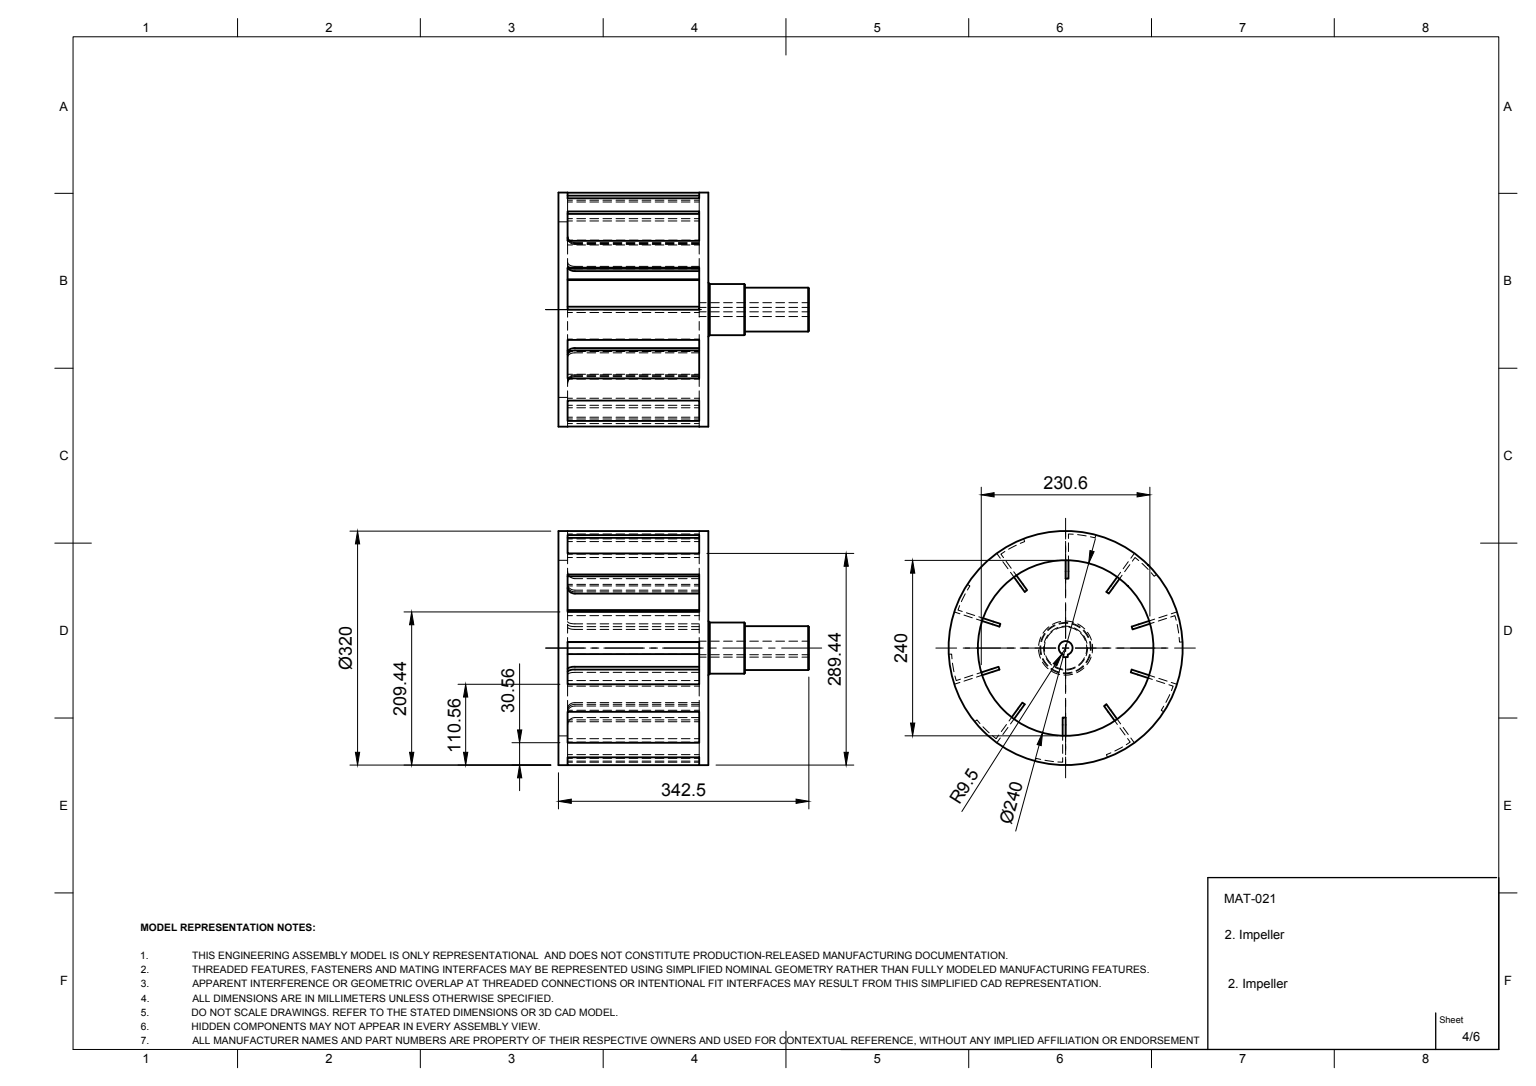
ISO-10303-21;
HEADER;
/* Generated by software containing ST-Developer
 * from STEP Tools, Inc. (www.steptools.com) 
 */

FILE_DESCRIPTION(
/* description */ ('STEP AP214'),
/* implementation_level */ '2;1');

FILE_NAME(
/* name */ '2. Impeller.step',
/* time_stamp */ '2026-11-14T06:27:21-08:00',
/* author */ (''),
/* organization */ (''),
/* preprocessor_version */ 'ST-DEVELOPER v20.2',
/* originating_system */ 'Autodesk Translation Framework v15.17.0.0',
/* authorisation */ '');

FILE_SCHEMA (('AUTOMOTIVE_DESIGN { 1 0 10303 214 3 1 1 }'));
ENDSEC;

DATA;
#10=MECHANICAL_DESIGN_GEOMETRIC_PRESENTATION_REPRESENTATION('',(#36),#27541);
#28=SHAPE_REPRESENTATION_RELATIONSHIP('SRR','None',#27562,#32);
#32=ADVANCED_BREP_SHAPE_REPRESENTATION('',(#63),#27538);
#36=STYLED_ITEM('',(#27591),#63);
#63=MANIFOLD_SOLID_BREP('Body1',#11824);
#248=PLANE('',#12491);
#249=PLANE('',#12492);
#250=PLANE('',#12493);
#251=PLANE('',#12494);
#252=PLANE('',#12495);
#253=PLANE('',#12496);
#254=PLANE('',#12497);
#255=PLANE('',#12498);
#256=PLANE('',#12499);
#257=PLANE('',#12500);
#258=PLANE('',#12501);
#259=PLANE('',#12512);
#260=PLANE('',#12513);
#261=PLANE('',#12514);
#262=PLANE('',#12515);
#263=PLANE('',#12516);
#264=PLANE('',#12520);
#265=PLANE('',#12521);
#266=PLANE('',#12524);
#267=PLANE('',#12525);
#268=PLANE('',#12529);
#269=PLANE('',#12530);
#270=PLANE('',#12532);
#271=PLANE('',#12533);
#272=PLANE('',#12537);
#273=PLANE('',#12538);
#274=PLANE('',#12540);
#275=PLANE('',#12541);
#276=PLANE('',#12545);
#277=PLANE('',#12546);
#278=PLANE('',#12548);
#279=PLANE('',#12549);
#280=PLANE('',#12553);
#281=PLANE('',#12554);
#282=PLANE('',#12556);
#283=PLANE('',#12557);
#284=PLANE('',#12561);
#285=PLANE('',#12562);
#286=PLANE('',#12564);
#287=PLANE('',#12565);
#288=PLANE('',#12569);
#289=PLANE('',#12570);
#290=PLANE('',#12572);
#291=PLANE('',#12573);
#292=PLANE('',#12577);
#293=PLANE('',#12578);
#294=PLANE('',#12580);
#295=PLANE('',#12581);
#296=PLANE('',#12585);
#297=PLANE('',#12586);
#298=PLANE('',#12588);
#299=PLANE('',#12589);
#300=PLANE('',#12593);
#301=PLANE('',#12594);
#302=PLANE('',#12605);
#303=PLANE('',#12606);
#304=PLANE('',#12607);
#305=PLANE('',#12608);
#306=PLANE('',#12609);
#307=PLANE('',#12610);
#308=PLANE('',#12611);
#309=PLANE('',#12612);
#310=PLANE('',#12613);
#311=PLANE('',#12614);
#312=PLANE('',#12615);
#313=PLANE('',#12616);
#314=PLANE('',#12617);
#315=PLANE('',#12618);
#569=FACE_BOUND('',#1666,.T.);
#570=FACE_BOUND('',#1667,.T.);
#571=FACE_BOUND('',#1668,.T.);
#572=FACE_BOUND('',#1669,.T.);
#573=FACE_BOUND('',#1670,.T.);
#574=FACE_BOUND('',#1671,.T.);
#575=FACE_BOUND('',#1672,.T.);
#576=FACE_BOUND('',#1673,.T.);
#577=FACE_BOUND('',#1674,.T.);
#578=FACE_BOUND('',#1688,.T.);
#579=FACE_BOUND('',#1690,.T.);
#580=FACE_BOUND('',#1692,.T.);
#581=FACE_BOUND('',#1694,.T.);
#582=FACE_BOUND('',#1766,.T.);
#625=CONICAL_SURFACE('',#12425,37.0000000000001,0.78539816339744);
#626=CONICAL_SURFACE('',#12429,30.,0.785398163397422);
#627=CONICAL_SURFACE('',#12433,35.,0.785398163397445);
#952=FACE_OUTER_BOUND('',#1660,.T.);
#953=FACE_OUTER_BOUND('',#1661,.T.);
#954=FACE_OUTER_BOUND('',#1662,.T.);
#955=FACE_OUTER_BOUND('',#1663,.T.);
#956=FACE_OUTER_BOUND('',#1664,.T.);
#957=FACE_OUTER_BOUND('',#1665,.T.);
#958=FACE_OUTER_BOUND('',#1675,.T.);
#959=FACE_OUTER_BOUND('',#1676,.T.);
#960=FACE_OUTER_BOUND('',#1677,.T.);
#961=FACE_OUTER_BOUND('',#1678,.T.);
#962=FACE_OUTER_BOUND('',#1679,.T.);
#963=FACE_OUTER_BOUND('',#1680,.T.);
#964=FACE_OUTER_BOUND('',#1681,.T.);
#965=FACE_OUTER_BOUND('',#1682,.T.);
#966=FACE_OUTER_BOUND('',#1683,.T.);
#967=FACE_OUTER_BOUND('',#1684,.T.);
#968=FACE_OUTER_BOUND('',#1685,.T.);
#969=FACE_OUTER_BOUND('',#1686,.T.);
#970=FACE_OUTER_BOUND('',#1687,.T.);
#971=FACE_OUTER_BOUND('',#1689,.T.);
#972=FACE_OUTER_BOUND('',#1691,.T.);
#973=FACE_OUTER_BOUND('',#1693,.T.);
#974=FACE_OUTER_BOUND('',#1695,.T.);
#975=FACE_OUTER_BOUND('',#1696,.T.);
#976=FACE_OUTER_BOUND('',#1697,.T.);
#977=FACE_OUTER_BOUND('',#1698,.T.);
#978=FACE_OUTER_BOUND('',#1699,.T.);
#979=FACE_OUTER_BOUND('',#1700,.T.);
#980=FACE_OUTER_BOUND('',#1701,.T.);
#981=FACE_OUTER_BOUND('',#1702,.T.);
#982=FACE_OUTER_BOUND('',#1703,.T.);
#983=FACE_OUTER_BOUND('',#1704,.T.);
#984=FACE_OUTER_BOUND('',#1705,.T.);
#985=FACE_OUTER_BOUND('',#1706,.T.);
#986=FACE_OUTER_BOUND('',#1707,.T.);
#987=FACE_OUTER_BOUND('',#1708,.T.);
#988=FACE_OUTER_BOUND('',#1709,.T.);
#989=FACE_OUTER_BOUND('',#1710,.T.);
#990=FACE_OUTER_BOUND('',#1711,.T.);
#991=FACE_OUTER_BOUND('',#1712,.T.);
#992=FACE_OUTER_BOUND('',#1713,.T.);
#993=FACE_OUTER_BOUND('',#1714,.T.);
#994=FACE_OUTER_BOUND('',#1715,.T.);
#995=FACE_OUTER_BOUND('',#1716,.T.);
#996=FACE_OUTER_BOUND('',#1717,.T.);
#997=FACE_OUTER_BOUND('',#1718,.T.);
#998=FACE_OUTER_BOUND('',#1719,.T.);
#999=FACE_OUTER_BOUND('',#1720,.T.);
#1000=FACE_OUTER_BOUND('',#1721,.T.);
#1001=FACE_OUTER_BOUND('',#1722,.T.);
#1002=FACE_OUTER_BOUND('',#1723,.T.);
#1003=FACE_OUTER_BOUND('',#1724,.T.);
#1004=FACE_OUTER_BOUND('',#1725,.T.);
#1005=FACE_OUTER_BOUND('',#1726,.T.);
#1006=FACE_OUTER_BOUND('',#1727,.T.);
#1007=FACE_OUTER_BOUND('',#1728,.T.);
#1008=FACE_OUTER_BOUND('',#1729,.T.);
#1009=FACE_OUTER_BOUND('',#1730,.T.);
#1010=FACE_OUTER_BOUND('',#1731,.T.);
#1011=FACE_OUTER_BOUND('',#1732,.T.);
#1012=FACE_OUTER_BOUND('',#1733,.T.);
#1013=FACE_OUTER_BOUND('',#1734,.T.);
#1014=FACE_OUTER_BOUND('',#1735,.T.);
#1015=FACE_OUTER_BOUND('',#1736,.T.);
#1016=FACE_OUTER_BOUND('',#1737,.T.);
#1017=FACE_OUTER_BOUND('',#1738,.T.);
#1018=FACE_OUTER_BOUND('',#1739,.T.);
#1019=FACE_OUTER_BOUND('',#1740,.T.);
#1020=FACE_OUTER_BOUND('',#1741,.T.);
#1021=FACE_OUTER_BOUND('',#1742,.T.);
#1022=FACE_OUTER_BOUND('',#1743,.T.);
#1023=FACE_OUTER_BOUND('',#1744,.T.);
#1024=FACE_OUTER_BOUND('',#1745,.T.);
#1025=FACE_OUTER_BOUND('',#1746,.T.);
#1026=FACE_OUTER_BOUND('',#1747,.T.);
#1027=FACE_OUTER_BOUND('',#1748,.T.);
#1028=FACE_OUTER_BOUND('',#1749,.T.);
#1029=FACE_OUTER_BOUND('',#1750,.T.);
#1030=FACE_OUTER_BOUND('',#1751,.T.);
#1031=FACE_OUTER_BOUND('',#1752,.T.);
#1032=FACE_OUTER_BOUND('',#1753,.T.);
#1033=FACE_OUTER_BOUND('',#1754,.T.);
#1034=FACE_OUTER_BOUND('',#1755,.T.);
#1035=FACE_OUTER_BOUND('',#1756,.T.);
#1036=FACE_OUTER_BOUND('',#1757,.T.);
#1037=FACE_OUTER_BOUND('',#1758,.T.);
#1038=FACE_OUTER_BOUND('',#1759,.T.);
#1039=FACE_OUTER_BOUND('',#1760,.T.);
#1040=FACE_OUTER_BOUND('',#1761,.T.);
#1041=FACE_OUTER_BOUND('',#1762,.T.);
#1042=FACE_OUTER_BOUND('',#1763,.T.);
#1043=FACE_OUTER_BOUND('',#1764,.T.);
#1044=FACE_OUTER_BOUND('',#1765,.T.);
#1045=FACE_OUTER_BOUND('',#1767,.T.);
#1046=FACE_OUTER_BOUND('',#1768,.T.);
#1047=FACE_OUTER_BOUND('',#1769,.T.);
#1660=EDGE_LOOP('',(#8644,#8645,#8646,#8647,#8648));
#1661=EDGE_LOOP('',(#8649,#8650,#8651,#8652,#8653));
#1662=EDGE_LOOP('',(#8654,#8655,#8656,#8657,#8658));
#1663=EDGE_LOOP('',(#8659,#8660,#8661,#8662));
#1664=EDGE_LOOP('',(#8663,#8664,#8665,#8666,#8667,#8668,#8669,#8670,#8671,
#8672,#8673,#8674,#8675,#8676,#8677,#8678,#8679,#8680,#8681,#8682,#8683,
#8684,#8685,#8686));
#1665=EDGE_LOOP('',(#8687,#8688,#8689,#8690,#8691,#8692,#8693,#8694,#8695,
#8696,#8697,#8698));
#1666=EDGE_LOOP('',(#8699,#8700,#8701,#8702));
#1667=EDGE_LOOP('',(#8703,#8704,#8705,#8706));
#1668=EDGE_LOOP('',(#8707,#8708,#8709,#8710));
#1669=EDGE_LOOP('',(#8711,#8712,#8713,#8714));
#1670=EDGE_LOOP('',(#8715,#8716,#8717,#8718));
#1671=EDGE_LOOP('',(#8719,#8720,#8721,#8722));
#1672=EDGE_LOOP('',(#8723,#8724,#8725,#8726));
#1673=EDGE_LOOP('',(#8727,#8728,#8729,#8730));
#1674=EDGE_LOOP('',(#8731,#8732,#8733,#8734));
#1675=EDGE_LOOP('',(#8735,#8736,#8737,#8738,#8739,#8740));
#1676=EDGE_LOOP('',(#8741,#8742,#8743,#8744,#8745));
#1677=EDGE_LOOP('',(#8746,#8747,#8748,#8749));
#1678=EDGE_LOOP('',(#8750,#8751,#8752,#8753));
#1679=EDGE_LOOP('',(#8754,#8755,#8756,#8757));
#1680=EDGE_LOOP('',(#8758,#8759,#8760,#8761));
#1681=EDGE_LOOP('',(#8762,#8763,#8764,#8765));
#1682=EDGE_LOOP('',(#8766,#8767,#8768,#8769));
#1683=EDGE_LOOP('',(#8770,#8771,#8772,#8773));
#1684=EDGE_LOOP('',(#8774,#8775,#8776,#8777));
#1685=EDGE_LOOP('',(#8778,#8779,#8780,#8781));
#1686=EDGE_LOOP('',(#8782,#8783,#8784,#8785));
#1687=EDGE_LOOP('',(#8786,#8787,#8788,#8789,#8790,#8791,#8792,#8793,#8794,
#8795,#8796,#8797,#8798,#8799,#8800,#8801,#8802,#8803,#8804,#8805,#8806,
#8807,#8808,#8809,#8810,#8811,#8812,#8813,#8814,#8815,#8816,#8817,#8818,
#8819,#8820,#8821,#8822,#8823,#8824,#8825,#8826,#8827,#8828,#8829,#8830,
#8831,#8832,#8833,#8834,#8835,#8836,#8837,#8838,#8839,#8840,#8841,#8842,
#8843,#8844,#8845,#8846));
#1688=EDGE_LOOP('',(#8847,#8848,#8849,#8850));
#1689=EDGE_LOOP('',(#8851));
#1690=EDGE_LOOP('',(#8852,#8853,#8854,#8855));
#1691=EDGE_LOOP('',(#8856));
#1692=EDGE_LOOP('',(#8857));
#1693=EDGE_LOOP('',(#8858));
#1694=EDGE_LOOP('',(#8859));
#1695=EDGE_LOOP('',(#8860,#8861,#8862,#8863));
#1696=EDGE_LOOP('',(#8864,#8865,#8866,#8867,#8868,#8869));
#1697=EDGE_LOOP('',(#8870,#8871,#8872,#8873));
#1698=EDGE_LOOP('',(#8874,#8875,#8876,#8877));
#1699=EDGE_LOOP('',(#8878,#8879,#8880,#8881,#8882,#8883));
#1700=EDGE_LOOP('',(#8884,#8885,#8886,#8887));
#1701=EDGE_LOOP('',(#8888,#8889,#8890,#8891));
#1702=EDGE_LOOP('',(#8892,#8893,#8894,#8895,#8896,#8897));
#1703=EDGE_LOOP('',(#8898,#8899,#8900,#8901));
#1704=EDGE_LOOP('',(#8902,#8903,#8904,#8905));
#1705=EDGE_LOOP('',(#8906,#8907,#8908,#8909,#8910,#8911));
#1706=EDGE_LOOP('',(#8912,#8913,#8914,#8915));
#1707=EDGE_LOOP('',(#8916,#8917,#8918,#8919,#8920,#8921));
#1708=EDGE_LOOP('',(#8922,#8923,#8924,#8925));
#1709=EDGE_LOOP('',(#8926,#8927,#8928,#8929));
#1710=EDGE_LOOP('',(#8930,#8931,#8932,#8933,#8934,#8935));
#1711=EDGE_LOOP('',(#8936,#8937,#8938,#8939));
#1712=EDGE_LOOP('',(#8940,#8941,#8942,#8943,#8944,#8945));
#1713=EDGE_LOOP('',(#8946,#8947,#8948,#8949));
#1714=EDGE_LOOP('',(#8950,#8951,#8952,#8953));
#1715=EDGE_LOOP('',(#8954,#8955,#8956,#8957,#8958,#8959));
#1716=EDGE_LOOP('',(#8960,#8961,#8962,#8963));
#1717=EDGE_LOOP('',(#8964,#8965,#8966,#8967,#8968,#8969));
#1718=EDGE_LOOP('',(#8970,#8971,#8972,#8973));
#1719=EDGE_LOOP('',(#8974,#8975,#8976,#8977));
#1720=EDGE_LOOP('',(#8978,#8979,#8980,#8981,#8982,#8983));
#1721=EDGE_LOOP('',(#8984,#8985,#8986,#8987));
#1722=EDGE_LOOP('',(#8988,#8989,#8990,#8991,#8992,#8993));
#1723=EDGE_LOOP('',(#8994,#8995,#8996,#8997));
#1724=EDGE_LOOP('',(#8998,#8999,#9000,#9001));
#1725=EDGE_LOOP('',(#9002,#9003,#9004,#9005,#9006,#9007));
#1726=EDGE_LOOP('',(#9008,#9009,#9010,#9011));
#1727=EDGE_LOOP('',(#9012,#9013,#9014,#9015,#9016,#9017));
#1728=EDGE_LOOP('',(#9018,#9019,#9020,#9021));
#1729=EDGE_LOOP('',(#9022,#9023,#9024,#9025));
#1730=EDGE_LOOP('',(#9026,#9027,#9028,#9029,#9030,#9031));
#1731=EDGE_LOOP('',(#9032,#9033,#9034,#9035));
#1732=EDGE_LOOP('',(#9036,#9037,#9038,#9039,#9040,#9041));
#1733=EDGE_LOOP('',(#9042,#9043,#9044,#9045));
#1734=EDGE_LOOP('',(#9046,#9047,#9048,#9049));
#1735=EDGE_LOOP('',(#9050,#9051,#9052,#9053,#9054,#9055));
#1736=EDGE_LOOP('',(#9056,#9057,#9058,#9059));
#1737=EDGE_LOOP('',(#9060,#9061,#9062,#9063,#9064,#9065));
#1738=EDGE_LOOP('',(#9066,#9067,#9068,#9069));
#1739=EDGE_LOOP('',(#9070,#9071,#9072,#9073));
#1740=EDGE_LOOP('',(#9074,#9075,#9076,#9077,#9078,#9079));
#1741=EDGE_LOOP('',(#9080,#9081,#9082,#9083));
#1742=EDGE_LOOP('',(#9084,#9085,#9086,#9087,#9088,#9089));
#1743=EDGE_LOOP('',(#9090,#9091,#9092,#9093));
#1744=EDGE_LOOP('',(#9094,#9095,#9096,#9097));
#1745=EDGE_LOOP('',(#9098,#9099,#9100,#9101,#9102,#9103));
#1746=EDGE_LOOP('',(#9104,#9105,#9106,#9107));
#1747=EDGE_LOOP('',(#9108,#9109,#9110,#9111));
#1748=EDGE_LOOP('',(#9112,#9113,#9114,#9115));
#1749=EDGE_LOOP('',(#9116,#9117,#9118,#9119));
#1750=EDGE_LOOP('',(#9120,#9121,#9122,#9123));
#1751=EDGE_LOOP('',(#9124,#9125,#9126,#9127));
#1752=EDGE_LOOP('',(#9128,#9129,#9130,#9131));
#1753=EDGE_LOOP('',(#9132,#9133,#9134,#9135));
#1754=EDGE_LOOP('',(#9136,#9137,#9138,#9139));
#1755=EDGE_LOOP('',(#9140,#9141,#9142,#9143,#9144,#9145));
#1756=EDGE_LOOP('',(#9146,#9147,#9148,#9149,#9150,#9151));
#1757=EDGE_LOOP('',(#9152,#9153,#9154,#9155,#9156,#9157));
#1758=EDGE_LOOP('',(#9158,#9159,#9160,#9161,#9162,#9163));
#1759=EDGE_LOOP('',(#9164,#9165,#9166,#9167,#9168,#9169));
#1760=EDGE_LOOP('',(#9170,#9171,#9172,#9173,#9174,#9175));
#1761=EDGE_LOOP('',(#9176,#9177,#9178,#9179,#9180,#9181));
#1762=EDGE_LOOP('',(#9182,#9183,#9184,#9185,#9186,#9187));
#1763=EDGE_LOOP('',(#9188,#9189,#9190,#9191,#9192,#9193,#9194,#9195));
#1764=EDGE_LOOP('',(#9196,#9197,#9198,#9199,#9200,#9201));
#1765=EDGE_LOOP('',(#9202));
#1766=EDGE_LOOP('',(#9203));
#1767=EDGE_LOOP('',(#9204,#9205,#9206,#9207));
#1768=EDGE_LOOP('',(#9208,#9209,#9210,#9211));
#1769=EDGE_LOOP('',(#9212,#9213,#9214,#9215));
#2446=CIRCLE('',#12426,37.0000000000001);
#2447=CIRCLE('',#12427,35.);
#2448=CIRCLE('',#12428,35.);
#2449=CIRCLE('',#12430,30.);
#2450=CIRCLE('',#12431,30.);
#2451=CIRCLE('',#12432,29.0000000000001);
#2452=CIRCLE('',#12434,35.);
#2453=CIRCLE('',#12435,35.);
#2454=CIRCLE('',#12436,34.0000000000001);
#2455=CIRCLE('',#12438,9.5);
#2456=CIRCLE('',#12439,9.5);
#2457=CIRCLE('',#12441,120.);
#2458=CIRCLE('',#12442,120.);
#2459=CIRCLE('',#12443,120.);
#2460=CIRCLE('',#12444,120.);
#2461=CIRCLE('',#12445,120.);
#2462=CIRCLE('',#12446,120.);
#2463=CIRCLE('',#12447,120.);
#2464=CIRCLE('',#12448,120.);
#2465=CIRCLE('',#12449,120.);
#2466=CIRCLE('',#12450,120.);
#2467=CIRCLE('',#12451,120.);
#2468=CIRCLE('',#12452,120.);
#2469=CIRCLE('',#12453,120.);
#2470=CIRCLE('',#12454,120.);
#2471=CIRCLE('',#12455,120.);
#2472=CIRCLE('',#12456,120.);
#2473=CIRCLE('',#12457,120.);
#2474=CIRCLE('',#12458,120.);
#2475=CIRCLE('',#12459,120.);
#2476=CIRCLE('',#12460,120.);
#2477=CIRCLE('',#12461,120.);
#2478=CIRCLE('',#12462,120.);
#2479=CIRCLE('',#12464,160.);
#2480=CIRCLE('',#12465,160.);
#2481=CIRCLE('',#12466,160.);
#2482=CIRCLE('',#12467,160.);
#2483=CIRCLE('',#12468,160.);
#2484=CIRCLE('',#12469,160.);
#2485=CIRCLE('',#12470,160.);
#2486=CIRCLE('',#12471,160.);
#2487=CIRCLE('',#12472,160.);
#2488=CIRCLE('',#12473,160.);
#2489=CIRCLE('',#12474,160.);
#2490=CIRCLE('',#12475,160.);
#2491=CIRCLE('',#12476,160.);
#2492=CIRCLE('',#12477,160.);
#2493=CIRCLE('',#12478,160.);
#2494=CIRCLE('',#12479,160.);
#2495=CIRCLE('',#12480,160.);
#2496=CIRCLE('',#12481,160.);
#2497=CIRCLE('',#12482,160.);
#2498=CIRCLE('',#12483,160.);
#2499=CIRCLE('',#12484,160.);
#2500=CIRCLE('',#12485,160.);
#2501=CIRCLE('',#12486,160.);
#2502=CIRCLE('',#12487,160.);
#2503=CIRCLE('',#12490,30.);
#2504=CIRCLE('',#12502,156.);
#2505=CIRCLE('',#12503,156.);
#2506=CIRCLE('',#12504,156.);
#2507=CIRCLE('',#12505,156.);
#2508=CIRCLE('',#12506,156.);
#2509=CIRCLE('',#12507,156.);
#2510=CIRCLE('',#12508,156.);
#2511=CIRCLE('',#12509,156.);
#2512=CIRCLE('',#12510,156.);
#2513=CIRCLE('',#12511,156.);
#2514=CIRCLE('',#12517,10.);
#2515=CIRCLE('',#12519,156.);
#2516=CIRCLE('',#12522,10.);
#2517=CIRCLE('',#12526,10.);
#2518=CIRCLE('',#12528,156.);
#2519=CIRCLE('',#12531,10.);
#2520=CIRCLE('',#12534,10.);
#2521=CIRCLE('',#12536,156.);
#2522=CIRCLE('',#12539,10.);
#2523=CIRCLE('',#12542,10.);
#2524=CIRCLE('',#12544,156.);
#2525=CIRCLE('',#12547,10.);
#2526=CIRCLE('',#12550,10.);
#2527=CIRCLE('',#12552,156.);
#2528=CIRCLE('',#12555,10.);
#2529=CIRCLE('',#12558,10.);
#2530=CIRCLE('',#12560,156.);
#2531=CIRCLE('',#12563,10.);
#2532=CIRCLE('',#12566,10.);
#2533=CIRCLE('',#12568,156.);
#2534=CIRCLE('',#12571,10.);
#2535=CIRCLE('',#12574,10.);
#2536=CIRCLE('',#12576,156.);
#2537=CIRCLE('',#12579,10.);
#2538=CIRCLE('',#12582,10.);
#2539=CIRCLE('',#12584,156.);
#2540=CIRCLE('',#12587,10.);
#2541=CIRCLE('',#12590,10.);
#2542=CIRCLE('',#12592,156.);
#2543=CIRCLE('',#12595,10.);
#2932=LINE('',#25208,#3944);
#2933=LINE('',#25218,#3945);
#2934=LINE('',#25226,#3946);
#2935=LINE('',#25233,#3947);
#2936=LINE('',#25236,#3948);
#2937=LINE('',#25241,#3949);
#2938=LINE('',#25287,#3950);
#2939=LINE('',#25291,#3951);
#2940=LINE('',#25295,#3952);
#2941=LINE('',#25300,#3953);
#2942=LINE('',#25306,#3954);
#2943=LINE('',#25309,#3955);
#2944=LINE('',#25312,#3956);
#2945=LINE('',#25316,#3957);
#2946=LINE('',#25320,#3958);
#2947=LINE('',#25324,#3959);
#2948=LINE('',#25328,#3960);
#2949=LINE('',#25332,#3961);
#2950=LINE('',#25336,#3962);
#2951=LINE('',#25340,#3963);
#2952=LINE('',#25346,#3964);
#2953=LINE('',#25349,#3965);
#2954=LINE('',#25352,#3966);
#2955=LINE('',#25356,#3967);
#2956=LINE('',#25360,#3968);
#2957=LINE('',#25364,#3969);
#2958=LINE('',#25368,#3970);
#2959=LINE('',#25372,#3971);
#2960=LINE('',#25375,#3972);
#2961=LINE('',#25378,#3973);
#2962=LINE('',#25382,#3974);
#2963=LINE('',#25384,#3975);
#2964=LINE('',#25385,#3976);
#2965=LINE('',#25388,#3977);
#2966=LINE('',#25390,#3978);
#2967=LINE('',#25391,#3979);
#2968=LINE('',#25394,#3980);
#2969=LINE('',#25396,#3981);
#2970=LINE('',#25397,#3982);
#2971=LINE('',#25400,#3983);
#2972=LINE('',#25402,#3984);
#2973=LINE('',#25403,#3985);
#2974=LINE('',#25406,#3986);
#2975=LINE('',#25408,#3987);
#2976=LINE('',#25409,#3988);
#2977=LINE('',#25412,#3989);
#2978=LINE('',#25414,#3990);
#2979=LINE('',#25415,#3991);
#2980=LINE('',#25418,#3992);
#2981=LINE('',#25420,#3993);
#2982=LINE('',#25421,#3994);
#2983=LINE('',#25424,#3995);
#2984=LINE('',#25426,#3996);
#2985=LINE('',#25427,#3997);
#2986=LINE('',#25430,#3998);
#2987=LINE('',#25432,#3999);
#2988=LINE('',#25433,#4000);
#2989=LINE('',#25436,#4001);
#2990=LINE('',#25438,#4002);
#2991=LINE('',#25439,#4003);
#2992=LINE('',#25442,#4004);
#2993=LINE('',#25446,#4005);
#2994=LINE('',#25448,#4006);
#2995=LINE('',#25449,#4007);
#2996=LINE('',#25451,#4008);
#2997=LINE('',#25455,#4009);
#2998=LINE('',#25457,#4010);
#2999=LINE('',#25458,#4011);
#3000=LINE('',#25460,#4012);
#3001=LINE('',#25464,#4013);
#3002=LINE('',#25466,#4014);
#3003=LINE('',#25467,#4015);
#3004=LINE('',#25469,#4016);
#3005=LINE('',#25473,#4017);
#3006=LINE('',#25475,#4018);
#3007=LINE('',#25476,#4019);
#3008=LINE('',#25478,#4020);
#3009=LINE('',#25482,#4021);
#3010=LINE('',#25484,#4022);
#3011=LINE('',#25485,#4023);
#3012=LINE('',#25487,#4024);
#3013=LINE('',#25491,#4025);
#3014=LINE('',#25493,#4026);
#3015=LINE('',#25494,#4027);
#3016=LINE('',#25496,#4028);
#3017=LINE('',#25500,#4029);
#3018=LINE('',#25502,#4030);
#3019=LINE('',#25503,#4031);
#3020=LINE('',#25505,#4032);
#3021=LINE('',#25509,#4033);
#3022=LINE('',#25511,#4034);
#3023=LINE('',#25512,#4035);
#3024=LINE('',#25514,#4036);
#3025=LINE('',#25518,#4037);
#3026=LINE('',#25520,#4038);
#3027=LINE('',#25521,#4039);
#3028=LINE('',#25523,#4040);
#3029=LINE('',#25527,#4041);
#3030=LINE('',#25529,#4042);
#3031=LINE('',#25530,#4043);
#3032=LINE('',#25532,#4044);
#3033=LINE('',#25534,#4045);
#3034=LINE('',#25535,#4046);
#3035=LINE('',#25538,#4047);
#3036=LINE('',#25540,#4048);
#3037=LINE('',#25541,#4049);
#3038=LINE('',#25546,#4050);
#3039=LINE('',#25548,#4051);
#3040=LINE('',#25549,#4052);
#3041=LINE('',#25553,#4053);
#3042=LINE('',#25554,#4054);
#3043=LINE('',#25557,#4055);
#3044=LINE('',#25560,#4056);
#3045=LINE('',#25563,#4057);
#3046=LINE('',#25567,#4058);
#3047=LINE('',#25569,#4059);
#3048=LINE('',#25570,#4060);
#3049=LINE('',#25574,#4061);
#3050=LINE('',#25575,#4062);
#3051=LINE('',#25578,#4063);
#3052=LINE('',#25581,#4064);
#3053=LINE('',#25584,#4065);
#3054=LINE('',#25587,#4066);
#3055=LINE('',#25589,#4067);
#3056=LINE('',#25590,#4068);
#3057=LINE('',#25594,#4069);
#3058=LINE('',#25595,#4070);
#3059=LINE('',#25598,#4071);
#3060=LINE('',#25601,#4072);
#3061=LINE('',#25604,#4073);
#3062=LINE('',#25607,#4074);
#3063=LINE('',#25609,#4075);
#3064=LINE('',#25610,#4076);
#3065=LINE('',#25614,#4077);
#3066=LINE('',#25615,#4078);
#3067=LINE('',#25618,#4079);
#3068=LINE('',#25621,#4080);
#3069=LINE('',#25624,#4081);
#3070=LINE('',#25627,#4082);
#3071=LINE('',#25629,#4083);
#3072=LINE('',#25630,#4084);
#3073=LINE('',#25634,#4085);
#3074=LINE('',#25635,#4086);
#3075=LINE('',#25638,#4087);
#3076=LINE('',#25641,#4088);
#3077=LINE('',#25644,#4089);
#3078=LINE('',#25647,#4090);
#3079=LINE('',#25649,#4091);
#3080=LINE('',#25650,#4092);
#3081=LINE('',#25654,#4093);
#3082=LINE('',#25655,#4094);
#3083=LINE('',#25658,#4095);
#3084=LINE('',#25661,#4096);
#3085=LINE('',#25664,#4097);
#3086=LINE('',#25667,#4098);
#3087=LINE('',#25669,#4099);
#3088=LINE('',#25670,#4100);
#3089=LINE('',#25674,#4101);
#3090=LINE('',#25675,#4102);
#3091=LINE('',#25678,#4103);
#3092=LINE('',#25681,#4104);
#3093=LINE('',#25684,#4105);
#3094=LINE('',#25687,#4106);
#3095=LINE('',#25689,#4107);
#3096=LINE('',#25690,#4108);
#3097=LINE('',#25694,#4109);
#3098=LINE('',#25695,#4110);
#3099=LINE('',#25698,#4111);
#3100=LINE('',#25701,#4112);
#3101=LINE('',#25704,#4113);
#3102=LINE('',#25707,#4114);
#3103=LINE('',#25709,#4115);
#3104=LINE('',#25710,#4116);
#3105=LINE('',#25714,#4117);
#3106=LINE('',#25715,#4118);
#3107=LINE('',#25718,#4119);
#3108=LINE('',#25721,#4120);
#3109=LINE('',#25724,#4121);
#3110=LINE('',#25727,#4122);
#3111=LINE('',#25729,#4123);
#3112=LINE('',#25730,#4124);
#3113=LINE('',#25734,#4125);
#3114=LINE('',#25735,#4126);
#3115=LINE('',#25738,#4127);
#3116=LINE('',#25741,#4128);
#3117=LINE('',#25744,#4129);
#3118=LINE('',#25766,#4130);
#3119=LINE('',#25768,#4131);
#3944=VECTOR('',#14429,37.0000000000001);
#3945=VECTOR('',#14440,30.);
#3946=VECTOR('',#14449,35.);
#3947=VECTOR('',#14456,1000.);
#3948=VECTOR('',#14459,1000.);
#3949=VECTOR('',#14464,120.);
#3950=VECTOR('',#14511,160.);
#3951=VECTOR('',#14514,1000.);
#3952=VECTOR('',#14517,160.);
#3953=VECTOR('',#14522,1000.);
#3954=VECTOR('',#14527,1000.);
#3955=VECTOR('',#14530,1000.);
#3956=VECTOR('',#14531,1000.);
#3957=VECTOR('',#14534,1000.);
#3958=VECTOR('',#14537,1000.);
#3959=VECTOR('',#14540,1000.);
#3960=VECTOR('',#14543,1000.);
#3961=VECTOR('',#14546,1000.);
#3962=VECTOR('',#14549,1000.);
#3963=VECTOR('',#14552,1000.);
#3964=VECTOR('',#14557,1000.);
#3965=VECTOR('',#14560,1000.);
#3966=VECTOR('',#14561,1000.);
#3967=VECTOR('',#14564,1000.);
#3968=VECTOR('',#14567,1000.);
#3969=VECTOR('',#14570,1000.);
#3970=VECTOR('',#14573,1000.);
#3971=VECTOR('',#14576,1000.);
#3972=VECTOR('',#14581,35.);
#3973=VECTOR('',#14584,30.);
#3974=VECTOR('',#14589,1000.);
#3975=VECTOR('',#14590,1000.);
#3976=VECTOR('',#14591,1000.);
#3977=VECTOR('',#14594,1000.);
#3978=VECTOR('',#14595,1000.);
#3979=VECTOR('',#14596,1000.);
#3980=VECTOR('',#14599,1000.);
#3981=VECTOR('',#14600,1000.);
#3982=VECTOR('',#14601,1000.);
#3983=VECTOR('',#14604,1000.);
#3984=VECTOR('',#14605,1000.);
#3985=VECTOR('',#14606,1000.);
#3986=VECTOR('',#14609,1000.);
#3987=VECTOR('',#14610,1000.);
#3988=VECTOR('',#14611,1000.);
#3989=VECTOR('',#14614,1000.);
#3990=VECTOR('',#14615,1000.);
#3991=VECTOR('',#14616,1000.);
#3992=VECTOR('',#14619,1000.);
#3993=VECTOR('',#14620,1000.);
#3994=VECTOR('',#14621,1000.);
#3995=VECTOR('',#14624,1000.);
#3996=VECTOR('',#14625,1000.);
#3997=VECTOR('',#14626,1000.);
#3998=VECTOR('',#14629,1000.);
#3999=VECTOR('',#14630,1000.);
#4000=VECTOR('',#14631,1000.);
#4001=VECTOR('',#14634,1000.);
#4002=VECTOR('',#14635,1000.);
#4003=VECTOR('',#14636,1000.);
#4004=VECTOR('',#14639,1000.);
#4005=VECTOR('',#14642,1000.);
#4006=VECTOR('',#14643,1000.);
#4007=VECTOR('',#14644,1000.);
#4008=VECTOR('',#14645,1000.);
#4009=VECTOR('',#14648,1000.);
#4010=VECTOR('',#14649,1000.);
#4011=VECTOR('',#14650,1000.);
#4012=VECTOR('',#14651,1000.);
#4013=VECTOR('',#14654,1000.);
#4014=VECTOR('',#14655,1000.);
#4015=VECTOR('',#14656,1000.);
#4016=VECTOR('',#14657,1000.);
#4017=VECTOR('',#14660,1000.);
#4018=VECTOR('',#14661,1000.);
#4019=VECTOR('',#14662,1000.);
#4020=VECTOR('',#14663,1000.);
#4021=VECTOR('',#14666,1000.);
#4022=VECTOR('',#14667,1000.);
#4023=VECTOR('',#14668,1000.);
#4024=VECTOR('',#14669,1000.);
#4025=VECTOR('',#14672,1000.);
#4026=VECTOR('',#14673,1000.);
#4027=VECTOR('',#14674,1000.);
#4028=VECTOR('',#14675,1000.);
#4029=VECTOR('',#14678,1000.);
#4030=VECTOR('',#14679,1000.);
#4031=VECTOR('',#14680,1000.);
#4032=VECTOR('',#14681,1000.);
#4033=VECTOR('',#14684,1000.);
#4034=VECTOR('',#14685,1000.);
#4035=VECTOR('',#14686,1000.);
#4036=VECTOR('',#14687,1000.);
#4037=VECTOR('',#14690,1000.);
#4038=VECTOR('',#14691,1000.);
#4039=VECTOR('',#14692,1000.);
#4040=VECTOR('',#14693,1000.);
#4041=VECTOR('',#14696,1000.);
#4042=VECTOR('',#14697,1000.);
#4043=VECTOR('',#14698,1000.);
#4044=VECTOR('',#14699,1000.);
#4045=VECTOR('',#14700,1000.);
#4046=VECTOR('',#14701,1000.);
#4047=VECTOR('',#14704,1000.);
#4048=VECTOR('',#14705,1000.);
#4049=VECTOR('',#14706,1000.);
#4050=VECTOR('',#14713,1000.);
#4051=VECTOR('',#14714,1000.);
#4052=VECTOR('',#14715,1000.);
#4053=VECTOR('',#14720,1000.);
#4054=VECTOR('',#14721,1000.);
#4055=VECTOR('',#14724,1000.);
#4056=VECTOR('',#14729,1000.);
#4057=VECTOR('',#14734,1000.);
#4058=VECTOR('',#14739,1000.);
#4059=VECTOR('',#14740,1000.);
#4060=VECTOR('',#14741,1000.);
#4061=VECTOR('',#14746,1000.);
#4062=VECTOR('',#14747,1000.);
#4063=VECTOR('',#14750,1000.);
#4064=VECTOR('',#14755,1000.);
#4065=VECTOR('',#14760,1000.);
#4066=VECTOR('',#14763,1000.);
#4067=VECTOR('',#14764,1000.);
#4068=VECTOR('',#14765,1000.);
#4069=VECTOR('',#14770,1000.);
#4070=VECTOR('',#14771,1000.);
#4071=VECTOR('',#14774,1000.);
#4072=VECTOR('',#14779,1000.);
#4073=VECTOR('',#14784,1000.);
#4074=VECTOR('',#14787,1000.);
#4075=VECTOR('',#14788,1000.);
#4076=VECTOR('',#14789,1000.);
#4077=VECTOR('',#14794,1000.);
#4078=VECTOR('',#14795,1000.);
#4079=VECTOR('',#14798,1000.);
#4080=VECTOR('',#14803,1000.);
#4081=VECTOR('',#14808,1000.);
#4082=VECTOR('',#14811,1000.);
#4083=VECTOR('',#14812,1000.);
#4084=VECTOR('',#14813,1000.);
#4085=VECTOR('',#14818,1000.);
#4086=VECTOR('',#14819,1000.);
#4087=VECTOR('',#14822,1000.);
#4088=VECTOR('',#14827,1000.);
#4089=VECTOR('',#14832,1000.);
#4090=VECTOR('',#14835,1000.);
#4091=VECTOR('',#14836,1000.);
#4092=VECTOR('',#14837,1000.);
#4093=VECTOR('',#14842,1000.);
#4094=VECTOR('',#14843,1000.);
#4095=VECTOR('',#14846,1000.);
#4096=VECTOR('',#14851,1000.);
#4097=VECTOR('',#14856,1000.);
#4098=VECTOR('',#14859,1000.);
#4099=VECTOR('',#14860,1000.);
#4100=VECTOR('',#14861,1000.);
#4101=VECTOR('',#14866,1000.);
#4102=VECTOR('',#14867,1000.);
#4103=VECTOR('',#14870,1000.);
#4104=VECTOR('',#14875,1000.);
#4105=VECTOR('',#14880,1000.);
#4106=VECTOR('',#14883,1000.);
#4107=VECTOR('',#14884,1000.);
#4108=VECTOR('',#14885,1000.);
#4109=VECTOR('',#14890,1000.);
#4110=VECTOR('',#14891,1000.);
#4111=VECTOR('',#14894,1000.);
#4112=VECTOR('',#14899,1000.);
#4113=VECTOR('',#14904,1000.);
#4114=VECTOR('',#14907,1000.);
#4115=VECTOR('',#14908,1000.);
#4116=VECTOR('',#14909,1000.);
#4117=VECTOR('',#14914,1000.);
#4118=VECTOR('',#14915,1000.);
#4119=VECTOR('',#14918,1000.);
#4120=VECTOR('',#14923,1000.);
#4121=VECTOR('',#14928,1000.);
#4122=VECTOR('',#14931,1000.);
#4123=VECTOR('',#14932,1000.);
#4124=VECTOR('',#14933,1000.);
#4125=VECTOR('',#14938,1000.);
#4126=VECTOR('',#14939,1000.);
#4127=VECTOR('',#14942,1000.);
#4128=VECTOR('',#14947,1000.);
#4129=VECTOR('',#14952,1000.);
#4130=VECTOR('',#14995,1000.);
#4131=VECTOR('',#14998,1000.);
#5082=VERTEX_POINT('',#25205);
#5083=VERTEX_POINT('',#25207);
#5084=VERTEX_POINT('',#25209);
#5085=VERTEX_POINT('',#25213);
#5086=VERTEX_POINT('',#25214);
#5087=VERTEX_POINT('',#25217);
#5088=VERTEX_POINT('',#25221);
#5089=VERTEX_POINT('',#25222);
#5090=VERTEX_POINT('',#25225);
#5091=VERTEX_POINT('',#25229);
#5092=VERTEX_POINT('',#25230);
#5093=VERTEX_POINT('',#25232);
#5094=VERTEX_POINT('',#25234);
#5095=VERTEX_POINT('',#25238);
#5096=VERTEX_POINT('',#25240);
#5097=VERTEX_POINT('',#25242);
#5098=VERTEX_POINT('',#25244);
#5099=VERTEX_POINT('',#25246);
#5100=VERTEX_POINT('',#25248);
#5101=VERTEX_POINT('',#25250);
#5102=VERTEX_POINT('',#25252);
#5103=VERTEX_POINT('',#25254);
#5104=VERTEX_POINT('',#25256);
#5105=VERTEX_POINT('',#25258);
#5106=VERTEX_POINT('',#25260);
#5107=VERTEX_POINT('',#25262);
#5108=VERTEX_POINT('',#25264);
#5109=VERTEX_POINT('',#25266);
#5110=VERTEX_POINT('',#25268);
#5111=VERTEX_POINT('',#25270);
#5112=VERTEX_POINT('',#25272);
#5113=VERTEX_POINT('',#25274);
#5114=VERTEX_POINT('',#25276);
#5115=VERTEX_POINT('',#25278);
#5116=VERTEX_POINT('',#25280);
#5117=VERTEX_POINT('',#25284);
#5118=VERTEX_POINT('',#25286);
#5119=VERTEX_POINT('',#25288);
#5120=VERTEX_POINT('',#25290);
#5121=VERTEX_POINT('',#25292);
#5122=VERTEX_POINT('',#25294);
#5123=VERTEX_POINT('',#25297);
#5124=VERTEX_POINT('',#25299);
#5125=VERTEX_POINT('',#25302);
#5126=VERTEX_POINT('',#25303);
#5127=VERTEX_POINT('',#25305);
#5128=VERTEX_POINT('',#25307);
#5129=VERTEX_POINT('',#25310);
#5130=VERTEX_POINT('',#25311);
#5131=VERTEX_POINT('',#25313);
#5132=VERTEX_POINT('',#25315);
#5133=VERTEX_POINT('',#25318);
#5134=VERTEX_POINT('',#25319);
#5135=VERTEX_POINT('',#25321);
#5136=VERTEX_POINT('',#25323);
#5137=VERTEX_POINT('',#25326);
#5138=VERTEX_POINT('',#25327);
#5139=VERTEX_POINT('',#25329);
#5140=VERTEX_POINT('',#25331);
#5141=VERTEX_POINT('',#25334);
#5142=VERTEX_POINT('',#25335);
#5143=VERTEX_POINT('',#25337);
#5144=VERTEX_POINT('',#25339);
#5145=VERTEX_POINT('',#25342);
#5146=VERTEX_POINT('',#25343);
#5147=VERTEX_POINT('',#25345);
#5148=VERTEX_POINT('',#25347);
#5149=VERTEX_POINT('',#25350);
#5150=VERTEX_POINT('',#25351);
#5151=VERTEX_POINT('',#25353);
#5152=VERTEX_POINT('',#25355);
#5153=VERTEX_POINT('',#25358);
#5154=VERTEX_POINT('',#25359);
#5155=VERTEX_POINT('',#25361);
#5156=VERTEX_POINT('',#25363);
#5157=VERTEX_POINT('',#25366);
#5158=VERTEX_POINT('',#25367);
#5159=VERTEX_POINT('',#25369);
#5160=VERTEX_POINT('',#25371);
#5161=VERTEX_POINT('',#25377);
#5162=VERTEX_POINT('',#25381);
#5163=VERTEX_POINT('',#25383);
#5164=VERTEX_POINT('',#25387);
#5165=VERTEX_POINT('',#25389);
#5166=VERTEX_POINT('',#25393);
#5167=VERTEX_POINT('',#25395);
#5168=VERTEX_POINT('',#25399);
#5169=VERTEX_POINT('',#25401);
#5170=VERTEX_POINT('',#25405);
#5171=VERTEX_POINT('',#25407);
#5172=VERTEX_POINT('',#25411);
#5173=VERTEX_POINT('',#25413);
#5174=VERTEX_POINT('',#25417);
#5175=VERTEX_POINT('',#25419);
#5176=VERTEX_POINT('',#25423);
#5177=VERTEX_POINT('',#25425);
#5178=VERTEX_POINT('',#25429);
#5179=VERTEX_POINT('',#25431);
#5180=VERTEX_POINT('',#25435);
#5181=VERTEX_POINT('',#25437);
#5182=VERTEX_POINT('',#25441);
#5183=VERTEX_POINT('',#25443);
#5184=VERTEX_POINT('',#25445);
#5185=VERTEX_POINT('',#25447);
#5186=VERTEX_POINT('',#25450);
#5187=VERTEX_POINT('',#25452);
#5188=VERTEX_POINT('',#25454);
#5189=VERTEX_POINT('',#25456);
#5190=VERTEX_POINT('',#25459);
#5191=VERTEX_POINT('',#25461);
#5192=VERTEX_POINT('',#25463);
#5193=VERTEX_POINT('',#25465);
#5194=VERTEX_POINT('',#25468);
#5195=VERTEX_POINT('',#25470);
#5196=VERTEX_POINT('',#25472);
#5197=VERTEX_POINT('',#25474);
#5198=VERTEX_POINT('',#25477);
#5199=VERTEX_POINT('',#25479);
#5200=VERTEX_POINT('',#25481);
#5201=VERTEX_POINT('',#25483);
#5202=VERTEX_POINT('',#25486);
#5203=VERTEX_POINT('',#25488);
#5204=VERTEX_POINT('',#25490);
#5205=VERTEX_POINT('',#25492);
#5206=VERTEX_POINT('',#25495);
#5207=VERTEX_POINT('',#25497);
#5208=VERTEX_POINT('',#25499);
#5209=VERTEX_POINT('',#25501);
#5210=VERTEX_POINT('',#25504);
#5211=VERTEX_POINT('',#25506);
#5212=VERTEX_POINT('',#25508);
#5213=VERTEX_POINT('',#25510);
#5214=VERTEX_POINT('',#25513);
#5215=VERTEX_POINT('',#25515);
#5216=VERTEX_POINT('',#25517);
#5217=VERTEX_POINT('',#25519);
#5218=VERTEX_POINT('',#25522);
#5219=VERTEX_POINT('',#25524);
#5220=VERTEX_POINT('',#25526);
#5221=VERTEX_POINT('',#25528);
#5222=VERTEX_POINT('',#25531);
#5223=VERTEX_POINT('',#25533);
#5224=VERTEX_POINT('',#25537);
#5225=VERTEX_POINT('',#25539);
#5226=VERTEX_POINT('',#25545);
#5227=VERTEX_POINT('',#25547);
#5228=VERTEX_POINT('',#25552);
#5229=VERTEX_POINT('',#25556);
#5230=VERTEX_POINT('',#25566);
#5231=VERTEX_POINT('',#25568);
#5232=VERTEX_POINT('',#25573);
#5233=VERTEX_POINT('',#25577);
#5234=VERTEX_POINT('',#25586);
#5235=VERTEX_POINT('',#25588);
#5236=VERTEX_POINT('',#25593);
#5237=VERTEX_POINT('',#25597);
#5238=VERTEX_POINT('',#25606);
#5239=VERTEX_POINT('',#25608);
#5240=VERTEX_POINT('',#25613);
#5241=VERTEX_POINT('',#25617);
#5242=VERTEX_POINT('',#25626);
#5243=VERTEX_POINT('',#25628);
#5244=VERTEX_POINT('',#25633);
#5245=VERTEX_POINT('',#25637);
#5246=VERTEX_POINT('',#25646);
#5247=VERTEX_POINT('',#25648);
#5248=VERTEX_POINT('',#25653);
#5249=VERTEX_POINT('',#25657);
#5250=VERTEX_POINT('',#25666);
#5251=VERTEX_POINT('',#25668);
#5252=VERTEX_POINT('',#25673);
#5253=VERTEX_POINT('',#25677);
#5254=VERTEX_POINT('',#25686);
#5255=VERTEX_POINT('',#25688);
#5256=VERTEX_POINT('',#25693);
#5257=VERTEX_POINT('',#25697);
#5258=VERTEX_POINT('',#25706);
#5259=VERTEX_POINT('',#25708);
#5260=VERTEX_POINT('',#25713);
#5261=VERTEX_POINT('',#25717);
#5262=VERTEX_POINT('',#25726);
#5263=VERTEX_POINT('',#25728);
#5264=VERTEX_POINT('',#25733);
#5265=VERTEX_POINT('',#25737);
#6390=EDGE_CURVE('',#5082,#5082,#2446,.T.);
#6391=EDGE_CURVE('',#5082,#5083,#2932,.T.);
#6392=EDGE_CURVE('',#5084,#5083,#2447,.T.);
#6393=EDGE_CURVE('',#5083,#5084,#2448,.T.);
#6394=EDGE_CURVE('',#5085,#5086,#2449,.T.);
#6395=EDGE_CURVE('',#5086,#5085,#2450,.T.);
#6396=EDGE_CURVE('',#5086,#5087,#2933,.T.);
#6397=EDGE_CURVE('',#5087,#5087,#2451,.T.);
#6398=EDGE_CURVE('',#5088,#5089,#2452,.T.);
#6399=EDGE_CURVE('',#5089,#5088,#2453,.T.);
#6400=EDGE_CURVE('',#5089,#5090,#2934,.T.);
#6401=EDGE_CURVE('',#5090,#5090,#2454,.T.);
#6402=EDGE_CURVE('',#5091,#5092,#2455,.T.);
#6403=EDGE_CURVE('',#5092,#5093,#2935,.T.);
#6404=EDGE_CURVE('',#5093,#5094,#2456,.T.);
#6405=EDGE_CURVE('',#5091,#5094,#2936,.T.);
#6406=EDGE_CURVE('',#5095,#5095,#2457,.T.);
#6407=EDGE_CURVE('',#5095,#5096,#2937,.T.);
#6408=EDGE_CURVE('',#5097,#5096,#2458,.T.);
#6409=EDGE_CURVE('',#5098,#5097,#2459,.T.);
#6410=EDGE_CURVE('',#5099,#5098,#2460,.T.);
#6411=EDGE_CURVE('',#5100,#5099,#2461,.T.);
#6412=EDGE_CURVE('',#5101,#5100,#2462,.T.);
#6413=EDGE_CURVE('',#5102,#5101,#2463,.T.);
#6414=EDGE_CURVE('',#5103,#5102,#2464,.T.);
#6415=EDGE_CURVE('',#5104,#5103,#2465,.T.);
#6416=EDGE_CURVE('',#5105,#5104,#2466,.T.);
#6417=EDGE_CURVE('',#5106,#5105,#2467,.T.);
#6418=EDGE_CURVE('',#5107,#5106,#2468,.T.);
#6419=EDGE_CURVE('',#5108,#5107,#2469,.T.);
#6420=EDGE_CURVE('',#5109,#5108,#2470,.T.);
#6421=EDGE_CURVE('',#5110,#5109,#2471,.T.);
#6422=EDGE_CURVE('',#5111,#5110,#2472,.T.);
#6423=EDGE_CURVE('',#5112,#5111,#2473,.T.);
#6424=EDGE_CURVE('',#5113,#5112,#2474,.T.);
#6425=EDGE_CURVE('',#5113,#5114,#2475,.T.);
#6426=EDGE_CURVE('',#5115,#5114,#2476,.T.);
#6427=EDGE_CURVE('',#5116,#5115,#2477,.T.);
#6428=EDGE_CURVE('',#5096,#5116,#2478,.T.);
#6429=EDGE_CURVE('',#5117,#5117,#2479,.T.);
#6430=EDGE_CURVE('',#5117,#5118,#2938,.T.);
#6431=EDGE_CURVE('',#5119,#5118,#2480,.T.);
#6432=EDGE_CURVE('',#5120,#5119,#2939,.T.);
#6433=EDGE_CURVE('',#5120,#5121,#2481,.T.);
#6434=EDGE_CURVE('',#5121,#5122,#2940,.T.);
#6435=EDGE_CURVE('',#5122,#5122,#2482,.T.);
#6436=EDGE_CURVE('',#5121,#5123,#2483,.T.);
#6437=EDGE_CURVE('',#5123,#5124,#2941,.T.);
#6438=EDGE_CURVE('',#5118,#5124,#2484,.T.);
#6439=EDGE_CURVE('',#5125,#5126,#2485,.T.);
#6440=EDGE_CURVE('',#5126,#5127,#2942,.T.);
#6441=EDGE_CURVE('',#5128,#5127,#2486,.T.);
#6442=EDGE_CURVE('',#5125,#5128,#2943,.T.);
#6443=EDGE_CURVE('',#5129,#5130,#2944,.T.);
#6444=EDGE_CURVE('',#5129,#5131,#2487,.T.);
#6445=EDGE_CURVE('',#5131,#5132,#2945,.T.);
#6446=EDGE_CURVE('',#5130,#5132,#2488,.T.);
#6447=EDGE_CURVE('',#5133,#5134,#2946,.T.);
#6448=EDGE_CURVE('',#5133,#5135,#2489,.T.);
#6449=EDGE_CURVE('',#5135,#5136,#2947,.T.);
#6450=EDGE_CURVE('',#5134,#5136,#2490,.T.);
#6451=EDGE_CURVE('',#5137,#5138,#2948,.T.);
#6452=EDGE_CURVE('',#5137,#5139,#2491,.T.);
#6453=EDGE_CURVE('',#5139,#5140,#2949,.T.);
#6454=EDGE_CURVE('',#5138,#5140,#2492,.T.);
#6455=EDGE_CURVE('',#5141,#5142,#2950,.T.);
#6456=EDGE_CURVE('',#5141,#5143,#2493,.T.);
#6457=EDGE_CURVE('',#5143,#5144,#2951,.T.);
#6458=EDGE_CURVE('',#5142,#5144,#2494,.T.);
#6459=EDGE_CURVE('',#5145,#5146,#2495,.T.);
#6460=EDGE_CURVE('',#5146,#5147,#2952,.T.);
#6461=EDGE_CURVE('',#5148,#5147,#2496,.T.);
#6462=EDGE_CURVE('',#5145,#5148,#2953,.T.);
#6463=EDGE_CURVE('',#5149,#5150,#2954,.T.);
#6464=EDGE_CURVE('',#5149,#5151,#2497,.T.);
#6465=EDGE_CURVE('',#5151,#5152,#2955,.T.);
#6466=EDGE_CURVE('',#5150,#5152,#2498,.T.);
#6467=EDGE_CURVE('',#5153,#5154,#2956,.T.);
#6468=EDGE_CURVE('',#5153,#5155,#2499,.T.);
#6469=EDGE_CURVE('',#5155,#5156,#2957,.T.);
#6470=EDGE_CURVE('',#5154,#5156,#2500,.T.);
#6471=EDGE_CURVE('',#5157,#5158,#2958,.T.);
#6472=EDGE_CURVE('',#5157,#5159,#2501,.T.);
#6473=EDGE_CURVE('',#5159,#5160,#2959,.T.);
#6474=EDGE_CURVE('',#5158,#5160,#2502,.T.);
#6475=EDGE_CURVE('',#5088,#5084,#2960,.T.);
#6476=EDGE_CURVE('',#5085,#5161,#2961,.T.);
#6477=EDGE_CURVE('',#5161,#5161,#2503,.T.);
#6478=EDGE_CURVE('',#5111,#5162,#2962,.T.);
#6479=EDGE_CURVE('',#5162,#5163,#2963,.T.);
#6480=EDGE_CURVE('',#5163,#5112,#2964,.T.);
#6481=EDGE_CURVE('',#5109,#5164,#2965,.T.);
#6482=EDGE_CURVE('',#5164,#5165,#2966,.T.);
#6483=EDGE_CURVE('',#5165,#5110,#2967,.T.);
#6484=EDGE_CURVE('',#5107,#5166,#2968,.T.);
#6485=EDGE_CURVE('',#5166,#5167,#2969,.T.);
#6486=EDGE_CURVE('',#5167,#5108,#2970,.T.);
#6487=EDGE_CURVE('',#5105,#5168,#2971,.T.);
#6488=EDGE_CURVE('',#5168,#5169,#2972,.T.);
#6489=EDGE_CURVE('',#5169,#5106,#2973,.T.);
#6490=EDGE_CURVE('',#5103,#5170,#2974,.T.);
#6491=EDGE_CURVE('',#5170,#5171,#2975,.T.);
#6492=EDGE_CURVE('',#5171,#5104,#2976,.T.);
#6493=EDGE_CURVE('',#5101,#5172,#2977,.T.);
#6494=EDGE_CURVE('',#5172,#5173,#2978,.T.);
#6495=EDGE_CURVE('',#5173,#5102,#2979,.T.);
#6496=EDGE_CURVE('',#5099,#5174,#2980,.T.);
#6497=EDGE_CURVE('',#5174,#5175,#2981,.T.);
#6498=EDGE_CURVE('',#5175,#5100,#2982,.T.);
#6499=EDGE_CURVE('',#5097,#5176,#2983,.T.);
#6500=EDGE_CURVE('',#5176,#5177,#2984,.T.);
#6501=EDGE_CURVE('',#5177,#5098,#2985,.T.);
#6502=EDGE_CURVE('',#5115,#5178,#2986,.T.);
#6503=EDGE_CURVE('',#5178,#5179,#2987,.T.);
#6504=EDGE_CURVE('',#5179,#5116,#2988,.T.);
#6505=EDGE_CURVE('',#5113,#5180,#2989,.T.);
#6506=EDGE_CURVE('',#5180,#5181,#2990,.T.);
#6507=EDGE_CURVE('',#5181,#5114,#2991,.T.);
#6508=EDGE_CURVE('',#5182,#5152,#2992,.T.);
#6509=EDGE_CURVE('',#5183,#5182,#2504,.T.);
#6510=EDGE_CURVE('',#5184,#5183,#2993,.T.);
#6511=EDGE_CURVE('',#5185,#5184,#2994,.T.);
#6512=EDGE_CURVE('',#5148,#5185,#2995,.T.);
#6513=EDGE_CURVE('',#5186,#5147,#2996,.T.);
#6514=EDGE_CURVE('',#5187,#5186,#2505,.T.);
#6515=EDGE_CURVE('',#5188,#5187,#2997,.T.);
#6516=EDGE_CURVE('',#5189,#5188,#2998,.T.);
#6517=EDGE_CURVE('',#5158,#5189,#2999,.T.);
#6518=EDGE_CURVE('',#5190,#5160,#3000,.T.);
#6519=EDGE_CURVE('',#5191,#5190,#2506,.T.);
#6520=EDGE_CURVE('',#5192,#5191,#3001,.T.);
#6521=EDGE_CURVE('',#5193,#5192,#3002,.T.);
#6522=EDGE_CURVE('',#5154,#5193,#3003,.T.);
#6523=EDGE_CURVE('',#5194,#5156,#3004,.T.);
#6524=EDGE_CURVE('',#5195,#5194,#2507,.T.);
#6525=EDGE_CURVE('',#5196,#5195,#3005,.T.);
#6526=EDGE_CURVE('',#5197,#5196,#3006,.T.);
#6527=EDGE_CURVE('',#5128,#5197,#3007,.T.);
#6528=EDGE_CURVE('',#5198,#5127,#3008,.T.);
#6529=EDGE_CURVE('',#5199,#5198,#2508,.T.);
#6530=EDGE_CURVE('',#5200,#5199,#3009,.T.);
#6531=EDGE_CURVE('',#5201,#5200,#3010,.T.);
#6532=EDGE_CURVE('',#5142,#5201,#3011,.T.);
#6533=EDGE_CURVE('',#5202,#5144,#3012,.T.);
#6534=EDGE_CURVE('',#5203,#5202,#2509,.T.);
#6535=EDGE_CURVE('',#5204,#5203,#3013,.T.);
#6536=EDGE_CURVE('',#5205,#5204,#3014,.T.);
#6537=EDGE_CURVE('',#5138,#5205,#3015,.T.);
#6538=EDGE_CURVE('',#5206,#5140,#3016,.T.);
#6539=EDGE_CURVE('',#5207,#5206,#2510,.T.);
#6540=EDGE_CURVE('',#5208,#5207,#3017,.T.);
#6541=EDGE_CURVE('',#5209,#5208,#3018,.T.);
#6542=EDGE_CURVE('',#5134,#5209,#3019,.T.);
#6543=EDGE_CURVE('',#5210,#5136,#3020,.T.);
#6544=EDGE_CURVE('',#5211,#5210,#2511,.T.);
#6545=EDGE_CURVE('',#5212,#5211,#3021,.T.);
#6546=EDGE_CURVE('',#5213,#5212,#3022,.T.);
#6547=EDGE_CURVE('',#5130,#5213,#3023,.T.);
#6548=EDGE_CURVE('',#5214,#5132,#3024,.T.);
#6549=EDGE_CURVE('',#5215,#5214,#2512,.T.);
#6550=EDGE_CURVE('',#5216,#5215,#3025,.T.);
#6551=EDGE_CURVE('',#5217,#5216,#3026,.T.);
#6552=EDGE_CURVE('',#5119,#5217,#3027,.T.);
#6553=EDGE_CURVE('',#5218,#5124,#3028,.T.);
#6554=EDGE_CURVE('',#5219,#5218,#2513,.T.);
#6555=EDGE_CURVE('',#5220,#5219,#3029,.T.);
#6556=EDGE_CURVE('',#5221,#5220,#3030,.T.);
#6557=EDGE_CURVE('',#5150,#5221,#3031,.T.);
#6558=EDGE_CURVE('',#5092,#5222,#3032,.T.);
#6559=EDGE_CURVE('',#5223,#5091,#3033,.T.);
#6560=EDGE_CURVE('',#5222,#5223,#3034,.T.);
#6561=EDGE_CURVE('',#5224,#5093,#3035,.T.);
#6562=EDGE_CURVE('',#5225,#5224,#3036,.T.);
#6563=EDGE_CURVE('',#5094,#5225,#3037,.T.);
#6564=EDGE_CURVE('',#5226,#5188,#3038,.T.);
#6565=EDGE_CURVE('',#5226,#5227,#3039,.T.);
#6566=EDGE_CURVE('',#5227,#5189,#3040,.T.);
#6567=EDGE_CURVE('',#5163,#5226,#2514,.T.);
#6568=EDGE_CURVE('',#5228,#5187,#3041,.T.);
#6569=EDGE_CURVE('',#5112,#5228,#3042,.T.);
#6570=EDGE_CURVE('',#5229,#5186,#3043,.T.);
#6571=EDGE_CURVE('',#5228,#5229,#2515,.T.);
#6572=EDGE_CURVE('',#5229,#5146,#3044,.T.);
#6573=EDGE_CURVE('',#5227,#5162,#2516,.T.);
#6574=EDGE_CURVE('',#5157,#5111,#3045,.T.);
#6575=EDGE_CURVE('',#5230,#5192,#3046,.T.);
#6576=EDGE_CURVE('',#5230,#5231,#3047,.T.);
#6577=EDGE_CURVE('',#5231,#5193,#3048,.T.);
#6578=EDGE_CURVE('',#5165,#5230,#2517,.T.);
#6579=EDGE_CURVE('',#5232,#5191,#3049,.T.);
#6580=EDGE_CURVE('',#5110,#5232,#3050,.T.);
#6581=EDGE_CURVE('',#5233,#5190,#3051,.T.);
#6582=EDGE_CURVE('',#5232,#5233,#2518,.T.);
#6583=EDGE_CURVE('',#5233,#5159,#3052,.T.);
#6584=EDGE_CURVE('',#5231,#5164,#2519,.T.);
#6585=EDGE_CURVE('',#5153,#5109,#3053,.T.);
#6586=EDGE_CURVE('',#5234,#5196,#3054,.T.);
#6587=EDGE_CURVE('',#5234,#5235,#3055,.T.);
#6588=EDGE_CURVE('',#5235,#5197,#3056,.T.);
#6589=EDGE_CURVE('',#5167,#5234,#2520,.T.);
#6590=EDGE_CURVE('',#5236,#5195,#3057,.T.);
#6591=EDGE_CURVE('',#5108,#5236,#3058,.T.);
#6592=EDGE_CURVE('',#5237,#5194,#3059,.T.);
#6593=EDGE_CURVE('',#5236,#5237,#2521,.T.);
#6594=EDGE_CURVE('',#5237,#5155,#3060,.T.);
#6595=EDGE_CURVE('',#5235,#5166,#2522,.T.);
#6596=EDGE_CURVE('',#5125,#5107,#3061,.T.);
#6597=EDGE_CURVE('',#5238,#5200,#3062,.T.);
#6598=EDGE_CURVE('',#5238,#5239,#3063,.T.);
#6599=EDGE_CURVE('',#5239,#5201,#3064,.T.);
#6600=EDGE_CURVE('',#5169,#5238,#2523,.T.);
#6601=EDGE_CURVE('',#5240,#5199,#3065,.T.);
#6602=EDGE_CURVE('',#5106,#5240,#3066,.T.);
#6603=EDGE_CURVE('',#5241,#5198,#3067,.T.);
#6604=EDGE_CURVE('',#5240,#5241,#2524,.T.);
#6605=EDGE_CURVE('',#5241,#5126,#3068,.T.);
#6606=EDGE_CURVE('',#5239,#5168,#2525,.T.);
#6607=EDGE_CURVE('',#5141,#5105,#3069,.T.);
#6608=EDGE_CURVE('',#5242,#5204,#3070,.T.);
#6609=EDGE_CURVE('',#5242,#5243,#3071,.T.);
#6610=EDGE_CURVE('',#5243,#5205,#3072,.T.);
#6611=EDGE_CURVE('',#5171,#5242,#2526,.T.);
#6612=EDGE_CURVE('',#5244,#5203,#3073,.T.);
#6613=EDGE_CURVE('',#5104,#5244,#3074,.T.);
#6614=EDGE_CURVE('',#5245,#5202,#3075,.T.);
#6615=EDGE_CURVE('',#5244,#5245,#2527,.T.);
#6616=EDGE_CURVE('',#5245,#5143,#3076,.T.);
#6617=EDGE_CURVE('',#5243,#5170,#2528,.T.);
#6618=EDGE_CURVE('',#5137,#5103,#3077,.T.);
#6619=EDGE_CURVE('',#5246,#5208,#3078,.T.);
#6620=EDGE_CURVE('',#5246,#5247,#3079,.T.);
#6621=EDGE_CURVE('',#5247,#5209,#3080,.T.);
#6622=EDGE_CURVE('',#5173,#5246,#2529,.T.);
#6623=EDGE_CURVE('',#5248,#5207,#3081,.T.);
#6624=EDGE_CURVE('',#5102,#5248,#3082,.T.);
#6625=EDGE_CURVE('',#5249,#5206,#3083,.T.);
#6626=EDGE_CURVE('',#5248,#5249,#2530,.T.);
#6627=EDGE_CURVE('',#5249,#5139,#3084,.T.);
#6628=EDGE_CURVE('',#5247,#5172,#2531,.T.);
#6629=EDGE_CURVE('',#5133,#5101,#3085,.T.);
#6630=EDGE_CURVE('',#5250,#5212,#3086,.T.);
#6631=EDGE_CURVE('',#5250,#5251,#3087,.T.);
#6632=EDGE_CURVE('',#5251,#5213,#3088,.T.);
#6633=EDGE_CURVE('',#5175,#5250,#2532,.T.);
#6634=EDGE_CURVE('',#5252,#5211,#3089,.T.);
#6635=EDGE_CURVE('',#5100,#5252,#3090,.T.);
#6636=EDGE_CURVE('',#5253,#5210,#3091,.T.);
#6637=EDGE_CURVE('',#5252,#5253,#2533,.T.);
#6638=EDGE_CURVE('',#5253,#5135,#3092,.T.);
#6639=EDGE_CURVE('',#5251,#5174,#2534,.T.);
#6640=EDGE_CURVE('',#5129,#5099,#3093,.T.);
#6641=EDGE_CURVE('',#5254,#5216,#3094,.T.);
#6642=EDGE_CURVE('',#5254,#5255,#3095,.T.);
#6643=EDGE_CURVE('',#5255,#5217,#3096,.T.);
#6644=EDGE_CURVE('',#5177,#5254,#2535,.T.);
#6645=EDGE_CURVE('',#5256,#5215,#3097,.T.);
#6646=EDGE_CURVE('',#5098,#5256,#3098,.T.);
#6647=EDGE_CURVE('',#5257,#5214,#3099,.T.);
#6648=EDGE_CURVE('',#5256,#5257,#2536,.T.);
#6649=EDGE_CURVE('',#5257,#5131,#3100,.T.);
#6650=EDGE_CURVE('',#5255,#5176,#2537,.T.);
#6651=EDGE_CURVE('',#5120,#5097,#3101,.T.);
#6652=EDGE_CURVE('',#5258,#5220,#3102,.T.);
#6653=EDGE_CURVE('',#5258,#5259,#3103,.T.);
#6654=EDGE_CURVE('',#5259,#5221,#3104,.T.);
#6655=EDGE_CURVE('',#5179,#5258,#2538,.T.);
#6656=EDGE_CURVE('',#5260,#5219,#3105,.T.);
#6657=EDGE_CURVE('',#5116,#5260,#3106,.T.);
#6658=EDGE_CURVE('',#5261,#5218,#3107,.T.);
#6659=EDGE_CURVE('',#5260,#5261,#2539,.T.);
#6660=EDGE_CURVE('',#5261,#5123,#3108,.T.);
#6661=EDGE_CURVE('',#5259,#5178,#2540,.T.);
#6662=EDGE_CURVE('',#5149,#5115,#3109,.T.);
#6663=EDGE_CURVE('',#5262,#5184,#3110,.T.);
#6664=EDGE_CURVE('',#5262,#5263,#3111,.T.);
#6665=EDGE_CURVE('',#5263,#5185,#3112,.T.);
#6666=EDGE_CURVE('',#5181,#5262,#2541,.T.);
#6667=EDGE_CURVE('',#5264,#5183,#3113,.T.);
#6668=EDGE_CURVE('',#5114,#5264,#3114,.T.);
#6669=EDGE_CURVE('',#5265,#5182,#3115,.T.);
#6670=EDGE_CURVE('',#5264,#5265,#2542,.T.);
#6671=EDGE_CURVE('',#5265,#5151,#3116,.T.);
#6672=EDGE_CURVE('',#5263,#5180,#2543,.T.);
#6673=EDGE_CURVE('',#5145,#5113,#3117,.T.);
#6674=EDGE_CURVE('',#5222,#5224,#3118,.T.);
#6675=EDGE_CURVE('',#5223,#5225,#3119,.T.);
#8644=ORIENTED_EDGE('',*,*,#6390,.F.);
#8645=ORIENTED_EDGE('',*,*,#6391,.T.);
#8646=ORIENTED_EDGE('',*,*,#6392,.F.);
#8647=ORIENTED_EDGE('',*,*,#6393,.F.);
#8648=ORIENTED_EDGE('',*,*,#6391,.F.);
#8649=ORIENTED_EDGE('',*,*,#6394,.F.);
#8650=ORIENTED_EDGE('',*,*,#6395,.F.);
#8651=ORIENTED_EDGE('',*,*,#6396,.T.);
#8652=ORIENTED_EDGE('',*,*,#6397,.F.);
#8653=ORIENTED_EDGE('',*,*,#6396,.F.);
#8654=ORIENTED_EDGE('',*,*,#6398,.F.);
#8655=ORIENTED_EDGE('',*,*,#6399,.F.);
#8656=ORIENTED_EDGE('',*,*,#6400,.T.);
#8657=ORIENTED_EDGE('',*,*,#6401,.F.);
#8658=ORIENTED_EDGE('',*,*,#6400,.F.);
#8659=ORIENTED_EDGE('',*,*,#6402,.T.);
#8660=ORIENTED_EDGE('',*,*,#6403,.T.);
#8661=ORIENTED_EDGE('',*,*,#6404,.T.);
#8662=ORIENTED_EDGE('',*,*,#6405,.F.);
#8663=ORIENTED_EDGE('',*,*,#6406,.T.);
#8664=ORIENTED_EDGE('',*,*,#6407,.T.);
#8665=ORIENTED_EDGE('',*,*,#6408,.F.);
#8666=ORIENTED_EDGE('',*,*,#6409,.F.);
#8667=ORIENTED_EDGE('',*,*,#6410,.F.);
#8668=ORIENTED_EDGE('',*,*,#6411,.F.);
#8669=ORIENTED_EDGE('',*,*,#6412,.F.);
#8670=ORIENTED_EDGE('',*,*,#6413,.F.);
#8671=ORIENTED_EDGE('',*,*,#6414,.F.);
#8672=ORIENTED_EDGE('',*,*,#6415,.F.);
#8673=ORIENTED_EDGE('',*,*,#6416,.F.);
#8674=ORIENTED_EDGE('',*,*,#6417,.F.);
#8675=ORIENTED_EDGE('',*,*,#6418,.F.);
#8676=ORIENTED_EDGE('',*,*,#6419,.F.);
#8677=ORIENTED_EDGE('',*,*,#6420,.F.);
#8678=ORIENTED_EDGE('',*,*,#6421,.F.);
#8679=ORIENTED_EDGE('',*,*,#6422,.F.);
#8680=ORIENTED_EDGE('',*,*,#6423,.F.);
#8681=ORIENTED_EDGE('',*,*,#6424,.F.);
#8682=ORIENTED_EDGE('',*,*,#6425,.T.);
#8683=ORIENTED_EDGE('',*,*,#6426,.F.);
#8684=ORIENTED_EDGE('',*,*,#6427,.F.);
#8685=ORIENTED_EDGE('',*,*,#6428,.F.);
#8686=ORIENTED_EDGE('',*,*,#6407,.F.);
#8687=ORIENTED_EDGE('',*,*,#6429,.T.);
#8688=ORIENTED_EDGE('',*,*,#6430,.T.);
#8689=ORIENTED_EDGE('',*,*,#6431,.F.);
#8690=ORIENTED_EDGE('',*,*,#6432,.F.);
#8691=ORIENTED_EDGE('',*,*,#6433,.T.);
#8692=ORIENTED_EDGE('',*,*,#6434,.T.);
#8693=ORIENTED_EDGE('',*,*,#6435,.F.);
#8694=ORIENTED_EDGE('',*,*,#6434,.F.);
#8695=ORIENTED_EDGE('',*,*,#6436,.T.);
#8696=ORIENTED_EDGE('',*,*,#6437,.T.);
#8697=ORIENTED_EDGE('',*,*,#6438,.F.);
#8698=ORIENTED_EDGE('',*,*,#6430,.F.);
#8699=ORIENTED_EDGE('',*,*,#6439,.T.);
#8700=ORIENTED_EDGE('',*,*,#6440,.T.);
#8701=ORIENTED_EDGE('',*,*,#6441,.F.);
#8702=ORIENTED_EDGE('',*,*,#6442,.F.);
#8703=ORIENTED_EDGE('',*,*,#6443,.F.);
#8704=ORIENTED_EDGE('',*,*,#6444,.T.);
#8705=ORIENTED_EDGE('',*,*,#6445,.T.);
#8706=ORIENTED_EDGE('',*,*,#6446,.F.);
#8707=ORIENTED_EDGE('',*,*,#6447,.F.);
#8708=ORIENTED_EDGE('',*,*,#6448,.T.);
#8709=ORIENTED_EDGE('',*,*,#6449,.T.);
#8710=ORIENTED_EDGE('',*,*,#6450,.F.);
#8711=ORIENTED_EDGE('',*,*,#6451,.F.);
#8712=ORIENTED_EDGE('',*,*,#6452,.T.);
#8713=ORIENTED_EDGE('',*,*,#6453,.T.);
#8714=ORIENTED_EDGE('',*,*,#6454,.F.);
#8715=ORIENTED_EDGE('',*,*,#6455,.F.);
#8716=ORIENTED_EDGE('',*,*,#6456,.T.);
#8717=ORIENTED_EDGE('',*,*,#6457,.T.);
#8718=ORIENTED_EDGE('',*,*,#6458,.F.);
#8719=ORIENTED_EDGE('',*,*,#6459,.T.);
#8720=ORIENTED_EDGE('',*,*,#6460,.T.);
#8721=ORIENTED_EDGE('',*,*,#6461,.F.);
#8722=ORIENTED_EDGE('',*,*,#6462,.F.);
#8723=ORIENTED_EDGE('',*,*,#6463,.F.);
#8724=ORIENTED_EDGE('',*,*,#6464,.T.);
#8725=ORIENTED_EDGE('',*,*,#6465,.T.);
#8726=ORIENTED_EDGE('',*,*,#6466,.F.);
#8727=ORIENTED_EDGE('',*,*,#6467,.F.);
#8728=ORIENTED_EDGE('',*,*,#6468,.T.);
#8729=ORIENTED_EDGE('',*,*,#6469,.T.);
#8730=ORIENTED_EDGE('',*,*,#6470,.F.);
#8731=ORIENTED_EDGE('',*,*,#6471,.F.);
#8732=ORIENTED_EDGE('',*,*,#6472,.T.);
#8733=ORIENTED_EDGE('',*,*,#6473,.T.);
#8734=ORIENTED_EDGE('',*,*,#6474,.F.);
#8735=ORIENTED_EDGE('',*,*,#6398,.T.);
#8736=ORIENTED_EDGE('',*,*,#6399,.T.);
#8737=ORIENTED_EDGE('',*,*,#6475,.T.);
#8738=ORIENTED_EDGE('',*,*,#6392,.T.);
#8739=ORIENTED_EDGE('',*,*,#6393,.T.);
#8740=ORIENTED_EDGE('',*,*,#6475,.F.);
#8741=ORIENTED_EDGE('',*,*,#6394,.T.);
#8742=ORIENTED_EDGE('',*,*,#6395,.T.);
#8743=ORIENTED_EDGE('',*,*,#6476,.T.);
#8744=ORIENTED_EDGE('',*,*,#6477,.F.);
#8745=ORIENTED_EDGE('',*,*,#6476,.F.);
#8746=ORIENTED_EDGE('',*,*,#6423,.T.);
#8747=ORIENTED_EDGE('',*,*,#6478,.T.);
#8748=ORIENTED_EDGE('',*,*,#6479,.T.);
#8749=ORIENTED_EDGE('',*,*,#6480,.T.);
#8750=ORIENTED_EDGE('',*,*,#6421,.T.);
#8751=ORIENTED_EDGE('',*,*,#6481,.T.);
#8752=ORIENTED_EDGE('',*,*,#6482,.T.);
#8753=ORIENTED_EDGE('',*,*,#6483,.T.);
#8754=ORIENTED_EDGE('',*,*,#6419,.T.);
#8755=ORIENTED_EDGE('',*,*,#6484,.T.);
#8756=ORIENTED_EDGE('',*,*,#6485,.T.);
#8757=ORIENTED_EDGE('',*,*,#6486,.T.);
#8758=ORIENTED_EDGE('',*,*,#6417,.T.);
#8759=ORIENTED_EDGE('',*,*,#6487,.T.);
#8760=ORIENTED_EDGE('',*,*,#6488,.T.);
#8761=ORIENTED_EDGE('',*,*,#6489,.T.);
#8762=ORIENTED_EDGE('',*,*,#6415,.T.);
#8763=ORIENTED_EDGE('',*,*,#6490,.T.);
#8764=ORIENTED_EDGE('',*,*,#6491,.T.);
#8765=ORIENTED_EDGE('',*,*,#6492,.T.);
#8766=ORIENTED_EDGE('',*,*,#6413,.T.);
#8767=ORIENTED_EDGE('',*,*,#6493,.T.);
#8768=ORIENTED_EDGE('',*,*,#6494,.T.);
#8769=ORIENTED_EDGE('',*,*,#6495,.T.);
#8770=ORIENTED_EDGE('',*,*,#6411,.T.);
#8771=ORIENTED_EDGE('',*,*,#6496,.T.);
#8772=ORIENTED_EDGE('',*,*,#6497,.T.);
#8773=ORIENTED_EDGE('',*,*,#6498,.T.);
#8774=ORIENTED_EDGE('',*,*,#6409,.T.);
#8775=ORIENTED_EDGE('',*,*,#6499,.T.);
#8776=ORIENTED_EDGE('',*,*,#6500,.T.);
#8777=ORIENTED_EDGE('',*,*,#6501,.T.);
#8778=ORIENTED_EDGE('',*,*,#6427,.T.);
#8779=ORIENTED_EDGE('',*,*,#6502,.T.);
#8780=ORIENTED_EDGE('',*,*,#6503,.T.);
#8781=ORIENTED_EDGE('',*,*,#6504,.T.);
#8782=ORIENTED_EDGE('',*,*,#6425,.F.);
#8783=ORIENTED_EDGE('',*,*,#6505,.T.);
#8784=ORIENTED_EDGE('',*,*,#6506,.T.);
#8785=ORIENTED_EDGE('',*,*,#6507,.T.);
#8786=ORIENTED_EDGE('',*,*,#6466,.T.);
#8787=ORIENTED_EDGE('',*,*,#6508,.F.);
#8788=ORIENTED_EDGE('',*,*,#6509,.F.);
#8789=ORIENTED_EDGE('',*,*,#6510,.F.);
#8790=ORIENTED_EDGE('',*,*,#6511,.F.);
#8791=ORIENTED_EDGE('',*,*,#6512,.F.);
#8792=ORIENTED_EDGE('',*,*,#6461,.T.);
#8793=ORIENTED_EDGE('',*,*,#6513,.F.);
#8794=ORIENTED_EDGE('',*,*,#6514,.F.);
#8795=ORIENTED_EDGE('',*,*,#6515,.F.);
#8796=ORIENTED_EDGE('',*,*,#6516,.F.);
#8797=ORIENTED_EDGE('',*,*,#6517,.F.);
#8798=ORIENTED_EDGE('',*,*,#6474,.T.);
#8799=ORIENTED_EDGE('',*,*,#6518,.F.);
#8800=ORIENTED_EDGE('',*,*,#6519,.F.);
#8801=ORIENTED_EDGE('',*,*,#6520,.F.);
#8802=ORIENTED_EDGE('',*,*,#6521,.F.);
#8803=ORIENTED_EDGE('',*,*,#6522,.F.);
#8804=ORIENTED_EDGE('',*,*,#6470,.T.);
#8805=ORIENTED_EDGE('',*,*,#6523,.F.);
#8806=ORIENTED_EDGE('',*,*,#6524,.F.);
#8807=ORIENTED_EDGE('',*,*,#6525,.F.);
#8808=ORIENTED_EDGE('',*,*,#6526,.F.);
#8809=ORIENTED_EDGE('',*,*,#6527,.F.);
#8810=ORIENTED_EDGE('',*,*,#6441,.T.);
#8811=ORIENTED_EDGE('',*,*,#6528,.F.);
#8812=ORIENTED_EDGE('',*,*,#6529,.F.);
#8813=ORIENTED_EDGE('',*,*,#6530,.F.);
#8814=ORIENTED_EDGE('',*,*,#6531,.F.);
#8815=ORIENTED_EDGE('',*,*,#6532,.F.);
#8816=ORIENTED_EDGE('',*,*,#6458,.T.);
#8817=ORIENTED_EDGE('',*,*,#6533,.F.);
#8818=ORIENTED_EDGE('',*,*,#6534,.F.);
#8819=ORIENTED_EDGE('',*,*,#6535,.F.);
#8820=ORIENTED_EDGE('',*,*,#6536,.F.);
#8821=ORIENTED_EDGE('',*,*,#6537,.F.);
#8822=ORIENTED_EDGE('',*,*,#6454,.T.);
#8823=ORIENTED_EDGE('',*,*,#6538,.F.);
#8824=ORIENTED_EDGE('',*,*,#6539,.F.);
#8825=ORIENTED_EDGE('',*,*,#6540,.F.);
#8826=ORIENTED_EDGE('',*,*,#6541,.F.);
#8827=ORIENTED_EDGE('',*,*,#6542,.F.);
#8828=ORIENTED_EDGE('',*,*,#6450,.T.);
#8829=ORIENTED_EDGE('',*,*,#6543,.F.);
#8830=ORIENTED_EDGE('',*,*,#6544,.F.);
#8831=ORIENTED_EDGE('',*,*,#6545,.F.);
#8832=ORIENTED_EDGE('',*,*,#6546,.F.);
#8833=ORIENTED_EDGE('',*,*,#6547,.F.);
#8834=ORIENTED_EDGE('',*,*,#6446,.T.);
#8835=ORIENTED_EDGE('',*,*,#6548,.F.);
#8836=ORIENTED_EDGE('',*,*,#6549,.F.);
#8837=ORIENTED_EDGE('',*,*,#6550,.F.);
#8838=ORIENTED_EDGE('',*,*,#6551,.F.);
#8839=ORIENTED_EDGE('',*,*,#6552,.F.);
#8840=ORIENTED_EDGE('',*,*,#6431,.T.);
#8841=ORIENTED_EDGE('',*,*,#6438,.T.);
#8842=ORIENTED_EDGE('',*,*,#6553,.F.);
#8843=ORIENTED_EDGE('',*,*,#6554,.F.);
#8844=ORIENTED_EDGE('',*,*,#6555,.F.);
#8845=ORIENTED_EDGE('',*,*,#6556,.F.);
#8846=ORIENTED_EDGE('',*,*,#6557,.F.);
#8847=ORIENTED_EDGE('',*,*,#6558,.F.);
#8848=ORIENTED_EDGE('',*,*,#6402,.F.);
#8849=ORIENTED_EDGE('',*,*,#6559,.F.);
#8850=ORIENTED_EDGE('',*,*,#6560,.F.);
#8851=ORIENTED_EDGE('',*,*,#6397,.T.);
#8852=ORIENTED_EDGE('',*,*,#6404,.F.);
#8853=ORIENTED_EDGE('',*,*,#6561,.F.);
#8854=ORIENTED_EDGE('',*,*,#6562,.F.);
#8855=ORIENTED_EDGE('',*,*,#6563,.F.);
#8856=ORIENTED_EDGE('',*,*,#6401,.T.);
#8857=ORIENTED_EDGE('',*,*,#6477,.T.);
#8858=ORIENTED_EDGE('',*,*,#6429,.F.);
#8859=ORIENTED_EDGE('',*,*,#6390,.T.);
#8860=ORIENTED_EDGE('',*,*,#6564,.F.);
#8861=ORIENTED_EDGE('',*,*,#6565,.T.);
#8862=ORIENTED_EDGE('',*,*,#6566,.T.);
#8863=ORIENTED_EDGE('',*,*,#6516,.T.);
#8864=ORIENTED_EDGE('',*,*,#6480,.F.);
#8865=ORIENTED_EDGE('',*,*,#6567,.T.);
#8866=ORIENTED_EDGE('',*,*,#6564,.T.);
#8867=ORIENTED_EDGE('',*,*,#6515,.T.);
#8868=ORIENTED_EDGE('',*,*,#6568,.F.);
#8869=ORIENTED_EDGE('',*,*,#6569,.F.);
#8870=ORIENTED_EDGE('',*,*,#6514,.T.);
#8871=ORIENTED_EDGE('',*,*,#6570,.F.);
#8872=ORIENTED_EDGE('',*,*,#6571,.F.);
#8873=ORIENTED_EDGE('',*,*,#6568,.T.);
#8874=ORIENTED_EDGE('',*,*,#6513,.T.);
#8875=ORIENTED_EDGE('',*,*,#6460,.F.);
#8876=ORIENTED_EDGE('',*,*,#6572,.F.);
#8877=ORIENTED_EDGE('',*,*,#6570,.T.);
#8878=ORIENTED_EDGE('',*,*,#6566,.F.);
#8879=ORIENTED_EDGE('',*,*,#6573,.T.);
#8880=ORIENTED_EDGE('',*,*,#6478,.F.);
#8881=ORIENTED_EDGE('',*,*,#6574,.F.);
#8882=ORIENTED_EDGE('',*,*,#6471,.T.);
#8883=ORIENTED_EDGE('',*,*,#6517,.T.);
#8884=ORIENTED_EDGE('',*,*,#6573,.F.);
#8885=ORIENTED_EDGE('',*,*,#6565,.F.);
#8886=ORIENTED_EDGE('',*,*,#6567,.F.);
#8887=ORIENTED_EDGE('',*,*,#6479,.F.);
#8888=ORIENTED_EDGE('',*,*,#6575,.F.);
#8889=ORIENTED_EDGE('',*,*,#6576,.T.);
#8890=ORIENTED_EDGE('',*,*,#6577,.T.);
#8891=ORIENTED_EDGE('',*,*,#6521,.T.);
#8892=ORIENTED_EDGE('',*,*,#6483,.F.);
#8893=ORIENTED_EDGE('',*,*,#6578,.T.);
#8894=ORIENTED_EDGE('',*,*,#6575,.T.);
#8895=ORIENTED_EDGE('',*,*,#6520,.T.);
#8896=ORIENTED_EDGE('',*,*,#6579,.F.);
#8897=ORIENTED_EDGE('',*,*,#6580,.F.);
#8898=ORIENTED_EDGE('',*,*,#6519,.T.);
#8899=ORIENTED_EDGE('',*,*,#6581,.F.);
#8900=ORIENTED_EDGE('',*,*,#6582,.F.);
#8901=ORIENTED_EDGE('',*,*,#6579,.T.);
#8902=ORIENTED_EDGE('',*,*,#6518,.T.);
#8903=ORIENTED_EDGE('',*,*,#6473,.F.);
#8904=ORIENTED_EDGE('',*,*,#6583,.F.);
#8905=ORIENTED_EDGE('',*,*,#6581,.T.);
#8906=ORIENTED_EDGE('',*,*,#6577,.F.);
#8907=ORIENTED_EDGE('',*,*,#6584,.T.);
#8908=ORIENTED_EDGE('',*,*,#6481,.F.);
#8909=ORIENTED_EDGE('',*,*,#6585,.F.);
#8910=ORIENTED_EDGE('',*,*,#6467,.T.);
#8911=ORIENTED_EDGE('',*,*,#6522,.T.);
#8912=ORIENTED_EDGE('',*,*,#6586,.F.);
#8913=ORIENTED_EDGE('',*,*,#6587,.T.);
#8914=ORIENTED_EDGE('',*,*,#6588,.T.);
#8915=ORIENTED_EDGE('',*,*,#6526,.T.);
#8916=ORIENTED_EDGE('',*,*,#6486,.F.);
#8917=ORIENTED_EDGE('',*,*,#6589,.T.);
#8918=ORIENTED_EDGE('',*,*,#6586,.T.);
#8919=ORIENTED_EDGE('',*,*,#6525,.T.);
#8920=ORIENTED_EDGE('',*,*,#6590,.F.);
#8921=ORIENTED_EDGE('',*,*,#6591,.F.);
#8922=ORIENTED_EDGE('',*,*,#6524,.T.);
#8923=ORIENTED_EDGE('',*,*,#6592,.F.);
#8924=ORIENTED_EDGE('',*,*,#6593,.F.);
#8925=ORIENTED_EDGE('',*,*,#6590,.T.);
#8926=ORIENTED_EDGE('',*,*,#6523,.T.);
#8927=ORIENTED_EDGE('',*,*,#6469,.F.);
#8928=ORIENTED_EDGE('',*,*,#6594,.F.);
#8929=ORIENTED_EDGE('',*,*,#6592,.T.);
#8930=ORIENTED_EDGE('',*,*,#6588,.F.);
#8931=ORIENTED_EDGE('',*,*,#6595,.T.);
#8932=ORIENTED_EDGE('',*,*,#6484,.F.);
#8933=ORIENTED_EDGE('',*,*,#6596,.F.);
#8934=ORIENTED_EDGE('',*,*,#6442,.T.);
#8935=ORIENTED_EDGE('',*,*,#6527,.T.);
#8936=ORIENTED_EDGE('',*,*,#6597,.F.);
#8937=ORIENTED_EDGE('',*,*,#6598,.T.);
#8938=ORIENTED_EDGE('',*,*,#6599,.T.);
#8939=ORIENTED_EDGE('',*,*,#6531,.T.);
#8940=ORIENTED_EDGE('',*,*,#6489,.F.);
#8941=ORIENTED_EDGE('',*,*,#6600,.T.);
#8942=ORIENTED_EDGE('',*,*,#6597,.T.);
#8943=ORIENTED_EDGE('',*,*,#6530,.T.);
#8944=ORIENTED_EDGE('',*,*,#6601,.F.);
#8945=ORIENTED_EDGE('',*,*,#6602,.F.);
#8946=ORIENTED_EDGE('',*,*,#6529,.T.);
#8947=ORIENTED_EDGE('',*,*,#6603,.F.);
#8948=ORIENTED_EDGE('',*,*,#6604,.F.);
#8949=ORIENTED_EDGE('',*,*,#6601,.T.);
#8950=ORIENTED_EDGE('',*,*,#6528,.T.);
#8951=ORIENTED_EDGE('',*,*,#6440,.F.);
#8952=ORIENTED_EDGE('',*,*,#6605,.F.);
#8953=ORIENTED_EDGE('',*,*,#6603,.T.);
#8954=ORIENTED_EDGE('',*,*,#6599,.F.);
#8955=ORIENTED_EDGE('',*,*,#6606,.T.);
#8956=ORIENTED_EDGE('',*,*,#6487,.F.);
#8957=ORIENTED_EDGE('',*,*,#6607,.F.);
#8958=ORIENTED_EDGE('',*,*,#6455,.T.);
#8959=ORIENTED_EDGE('',*,*,#6532,.T.);
#8960=ORIENTED_EDGE('',*,*,#6608,.F.);
#8961=ORIENTED_EDGE('',*,*,#6609,.T.);
#8962=ORIENTED_EDGE('',*,*,#6610,.T.);
#8963=ORIENTED_EDGE('',*,*,#6536,.T.);
#8964=ORIENTED_EDGE('',*,*,#6492,.F.);
#8965=ORIENTED_EDGE('',*,*,#6611,.T.);
#8966=ORIENTED_EDGE('',*,*,#6608,.T.);
#8967=ORIENTED_EDGE('',*,*,#6535,.T.);
#8968=ORIENTED_EDGE('',*,*,#6612,.F.);
#8969=ORIENTED_EDGE('',*,*,#6613,.F.);
#8970=ORIENTED_EDGE('',*,*,#6534,.T.);
#8971=ORIENTED_EDGE('',*,*,#6614,.F.);
#8972=ORIENTED_EDGE('',*,*,#6615,.F.);
#8973=ORIENTED_EDGE('',*,*,#6612,.T.);
#8974=ORIENTED_EDGE('',*,*,#6533,.T.);
#8975=ORIENTED_EDGE('',*,*,#6457,.F.);
#8976=ORIENTED_EDGE('',*,*,#6616,.F.);
#8977=ORIENTED_EDGE('',*,*,#6614,.T.);
#8978=ORIENTED_EDGE('',*,*,#6610,.F.);
#8979=ORIENTED_EDGE('',*,*,#6617,.T.);
#8980=ORIENTED_EDGE('',*,*,#6490,.F.);
#8981=ORIENTED_EDGE('',*,*,#6618,.F.);
#8982=ORIENTED_EDGE('',*,*,#6451,.T.);
#8983=ORIENTED_EDGE('',*,*,#6537,.T.);
#8984=ORIENTED_EDGE('',*,*,#6619,.F.);
#8985=ORIENTED_EDGE('',*,*,#6620,.T.);
#8986=ORIENTED_EDGE('',*,*,#6621,.T.);
#8987=ORIENTED_EDGE('',*,*,#6541,.T.);
#8988=ORIENTED_EDGE('',*,*,#6495,.F.);
#8989=ORIENTED_EDGE('',*,*,#6622,.T.);
#8990=ORIENTED_EDGE('',*,*,#6619,.T.);
#8991=ORIENTED_EDGE('',*,*,#6540,.T.);
#8992=ORIENTED_EDGE('',*,*,#6623,.F.);
#8993=ORIENTED_EDGE('',*,*,#6624,.F.);
#8994=ORIENTED_EDGE('',*,*,#6539,.T.);
#8995=ORIENTED_EDGE('',*,*,#6625,.F.);
#8996=ORIENTED_EDGE('',*,*,#6626,.F.);
#8997=ORIENTED_EDGE('',*,*,#6623,.T.);
#8998=ORIENTED_EDGE('',*,*,#6538,.T.);
#8999=ORIENTED_EDGE('',*,*,#6453,.F.);
#9000=ORIENTED_EDGE('',*,*,#6627,.F.);
#9001=ORIENTED_EDGE('',*,*,#6625,.T.);
#9002=ORIENTED_EDGE('',*,*,#6621,.F.);
#9003=ORIENTED_EDGE('',*,*,#6628,.T.);
#9004=ORIENTED_EDGE('',*,*,#6493,.F.);
#9005=ORIENTED_EDGE('',*,*,#6629,.F.);
#9006=ORIENTED_EDGE('',*,*,#6447,.T.);
#9007=ORIENTED_EDGE('',*,*,#6542,.T.);
#9008=ORIENTED_EDGE('',*,*,#6630,.F.);
#9009=ORIENTED_EDGE('',*,*,#6631,.T.);
#9010=ORIENTED_EDGE('',*,*,#6632,.T.);
#9011=ORIENTED_EDGE('',*,*,#6546,.T.);
#9012=ORIENTED_EDGE('',*,*,#6498,.F.);
#9013=ORIENTED_EDGE('',*,*,#6633,.T.);
#9014=ORIENTED_EDGE('',*,*,#6630,.T.);
#9015=ORIENTED_EDGE('',*,*,#6545,.T.);
#9016=ORIENTED_EDGE('',*,*,#6634,.F.);
#9017=ORIENTED_EDGE('',*,*,#6635,.F.);
#9018=ORIENTED_EDGE('',*,*,#6544,.T.);
#9019=ORIENTED_EDGE('',*,*,#6636,.F.);
#9020=ORIENTED_EDGE('',*,*,#6637,.F.);
#9021=ORIENTED_EDGE('',*,*,#6634,.T.);
#9022=ORIENTED_EDGE('',*,*,#6543,.T.);
#9023=ORIENTED_EDGE('',*,*,#6449,.F.);
#9024=ORIENTED_EDGE('',*,*,#6638,.F.);
#9025=ORIENTED_EDGE('',*,*,#6636,.T.);
#9026=ORIENTED_EDGE('',*,*,#6632,.F.);
#9027=ORIENTED_EDGE('',*,*,#6639,.T.);
#9028=ORIENTED_EDGE('',*,*,#6496,.F.);
#9029=ORIENTED_EDGE('',*,*,#6640,.F.);
#9030=ORIENTED_EDGE('',*,*,#6443,.T.);
#9031=ORIENTED_EDGE('',*,*,#6547,.T.);
#9032=ORIENTED_EDGE('',*,*,#6641,.F.);
#9033=ORIENTED_EDGE('',*,*,#6642,.T.);
#9034=ORIENTED_EDGE('',*,*,#6643,.T.);
#9035=ORIENTED_EDGE('',*,*,#6551,.T.);
#9036=ORIENTED_EDGE('',*,*,#6501,.F.);
#9037=ORIENTED_EDGE('',*,*,#6644,.T.);
#9038=ORIENTED_EDGE('',*,*,#6641,.T.);
#9039=ORIENTED_EDGE('',*,*,#6550,.T.);
#9040=ORIENTED_EDGE('',*,*,#6645,.F.);
#9041=ORIENTED_EDGE('',*,*,#6646,.F.);
#9042=ORIENTED_EDGE('',*,*,#6549,.T.);
#9043=ORIENTED_EDGE('',*,*,#6647,.F.);
#9044=ORIENTED_EDGE('',*,*,#6648,.F.);
#9045=ORIENTED_EDGE('',*,*,#6645,.T.);
#9046=ORIENTED_EDGE('',*,*,#6548,.T.);
#9047=ORIENTED_EDGE('',*,*,#6445,.F.);
#9048=ORIENTED_EDGE('',*,*,#6649,.F.);
#9049=ORIENTED_EDGE('',*,*,#6647,.T.);
#9050=ORIENTED_EDGE('',*,*,#6643,.F.);
#9051=ORIENTED_EDGE('',*,*,#6650,.T.);
#9052=ORIENTED_EDGE('',*,*,#6499,.F.);
#9053=ORIENTED_EDGE('',*,*,#6651,.F.);
#9054=ORIENTED_EDGE('',*,*,#6432,.T.);
#9055=ORIENTED_EDGE('',*,*,#6552,.T.);
#9056=ORIENTED_EDGE('',*,*,#6652,.F.);
#9057=ORIENTED_EDGE('',*,*,#6653,.T.);
#9058=ORIENTED_EDGE('',*,*,#6654,.T.);
#9059=ORIENTED_EDGE('',*,*,#6556,.T.);
#9060=ORIENTED_EDGE('',*,*,#6504,.F.);
#9061=ORIENTED_EDGE('',*,*,#6655,.T.);
#9062=ORIENTED_EDGE('',*,*,#6652,.T.);
#9063=ORIENTED_EDGE('',*,*,#6555,.T.);
#9064=ORIENTED_EDGE('',*,*,#6656,.F.);
#9065=ORIENTED_EDGE('',*,*,#6657,.F.);
#9066=ORIENTED_EDGE('',*,*,#6554,.T.);
#9067=ORIENTED_EDGE('',*,*,#6658,.F.);
#9068=ORIENTED_EDGE('',*,*,#6659,.F.);
#9069=ORIENTED_EDGE('',*,*,#6656,.T.);
#9070=ORIENTED_EDGE('',*,*,#6553,.T.);
#9071=ORIENTED_EDGE('',*,*,#6437,.F.);
#9072=ORIENTED_EDGE('',*,*,#6660,.F.);
#9073=ORIENTED_EDGE('',*,*,#6658,.T.);
#9074=ORIENTED_EDGE('',*,*,#6654,.F.);
#9075=ORIENTED_EDGE('',*,*,#6661,.T.);
#9076=ORIENTED_EDGE('',*,*,#6502,.F.);
#9077=ORIENTED_EDGE('',*,*,#6662,.F.);
#9078=ORIENTED_EDGE('',*,*,#6463,.T.);
#9079=ORIENTED_EDGE('',*,*,#6557,.T.);
#9080=ORIENTED_EDGE('',*,*,#6663,.F.);
#9081=ORIENTED_EDGE('',*,*,#6664,.T.);
#9082=ORIENTED_EDGE('',*,*,#6665,.T.);
#9083=ORIENTED_EDGE('',*,*,#6511,.T.);
#9084=ORIENTED_EDGE('',*,*,#6507,.F.);
#9085=ORIENTED_EDGE('',*,*,#6666,.T.);
#9086=ORIENTED_EDGE('',*,*,#6663,.T.);
#9087=ORIENTED_EDGE('',*,*,#6510,.T.);
#9088=ORIENTED_EDGE('',*,*,#6667,.F.);
#9089=ORIENTED_EDGE('',*,*,#6668,.F.);
#9090=ORIENTED_EDGE('',*,*,#6509,.T.);
#9091=ORIENTED_EDGE('',*,*,#6669,.F.);
#9092=ORIENTED_EDGE('',*,*,#6670,.F.);
#9093=ORIENTED_EDGE('',*,*,#6667,.T.);
#9094=ORIENTED_EDGE('',*,*,#6508,.T.);
#9095=ORIENTED_EDGE('',*,*,#6465,.F.);
#9096=ORIENTED_EDGE('',*,*,#6671,.F.);
#9097=ORIENTED_EDGE('',*,*,#6669,.T.);
#9098=ORIENTED_EDGE('',*,*,#6665,.F.);
#9099=ORIENTED_EDGE('',*,*,#6672,.T.);
#9100=ORIENTED_EDGE('',*,*,#6505,.F.);
#9101=ORIENTED_EDGE('',*,*,#6673,.F.);
#9102=ORIENTED_EDGE('',*,*,#6462,.T.);
#9103=ORIENTED_EDGE('',*,*,#6512,.T.);
#9104=ORIENTED_EDGE('',*,*,#6584,.F.);
#9105=ORIENTED_EDGE('',*,*,#6576,.F.);
#9106=ORIENTED_EDGE('',*,*,#6578,.F.);
#9107=ORIENTED_EDGE('',*,*,#6482,.F.);
#9108=ORIENTED_EDGE('',*,*,#6595,.F.);
#9109=ORIENTED_EDGE('',*,*,#6587,.F.);
#9110=ORIENTED_EDGE('',*,*,#6589,.F.);
#9111=ORIENTED_EDGE('',*,*,#6485,.F.);
#9112=ORIENTED_EDGE('',*,*,#6606,.F.);
#9113=ORIENTED_EDGE('',*,*,#6598,.F.);
#9114=ORIENTED_EDGE('',*,*,#6600,.F.);
#9115=ORIENTED_EDGE('',*,*,#6488,.F.);
#9116=ORIENTED_EDGE('',*,*,#6617,.F.);
#9117=ORIENTED_EDGE('',*,*,#6609,.F.);
#9118=ORIENTED_EDGE('',*,*,#6611,.F.);
#9119=ORIENTED_EDGE('',*,*,#6491,.F.);
#9120=ORIENTED_EDGE('',*,*,#6628,.F.);
#9121=ORIENTED_EDGE('',*,*,#6620,.F.);
#9122=ORIENTED_EDGE('',*,*,#6622,.F.);
#9123=ORIENTED_EDGE('',*,*,#6494,.F.);
#9124=ORIENTED_EDGE('',*,*,#6639,.F.);
#9125=ORIENTED_EDGE('',*,*,#6631,.F.);
#9126=ORIENTED_EDGE('',*,*,#6633,.F.);
#9127=ORIENTED_EDGE('',*,*,#6497,.F.);
#9128=ORIENTED_EDGE('',*,*,#6650,.F.);
#9129=ORIENTED_EDGE('',*,*,#6642,.F.);
#9130=ORIENTED_EDGE('',*,*,#6644,.F.);
#9131=ORIENTED_EDGE('',*,*,#6500,.F.);
#9132=ORIENTED_EDGE('',*,*,#6661,.F.);
#9133=ORIENTED_EDGE('',*,*,#6653,.F.);
#9134=ORIENTED_EDGE('',*,*,#6655,.F.);
#9135=ORIENTED_EDGE('',*,*,#6503,.F.);
#9136=ORIENTED_EDGE('',*,*,#6672,.F.);
#9137=ORIENTED_EDGE('',*,*,#6664,.F.);
#9138=ORIENTED_EDGE('',*,*,#6666,.F.);
#9139=ORIENTED_EDGE('',*,*,#6506,.F.);
#9140=ORIENTED_EDGE('',*,*,#6424,.T.);
#9141=ORIENTED_EDGE('',*,*,#6569,.T.);
#9142=ORIENTED_EDGE('',*,*,#6571,.T.);
#9143=ORIENTED_EDGE('',*,*,#6572,.T.);
#9144=ORIENTED_EDGE('',*,*,#6459,.F.);
#9145=ORIENTED_EDGE('',*,*,#6673,.T.);
#9146=ORIENTED_EDGE('',*,*,#6472,.F.);
#9147=ORIENTED_EDGE('',*,*,#6574,.T.);
#9148=ORIENTED_EDGE('',*,*,#6422,.T.);
#9149=ORIENTED_EDGE('',*,*,#6580,.T.);
#9150=ORIENTED_EDGE('',*,*,#6582,.T.);
#9151=ORIENTED_EDGE('',*,*,#6583,.T.);
#9152=ORIENTED_EDGE('',*,*,#6468,.F.);
#9153=ORIENTED_EDGE('',*,*,#6585,.T.);
#9154=ORIENTED_EDGE('',*,*,#6420,.T.);
#9155=ORIENTED_EDGE('',*,*,#6591,.T.);
#9156=ORIENTED_EDGE('',*,*,#6593,.T.);
#9157=ORIENTED_EDGE('',*,*,#6594,.T.);
#9158=ORIENTED_EDGE('',*,*,#6439,.F.);
#9159=ORIENTED_EDGE('',*,*,#6596,.T.);
#9160=ORIENTED_EDGE('',*,*,#6418,.T.);
#9161=ORIENTED_EDGE('',*,*,#6602,.T.);
#9162=ORIENTED_EDGE('',*,*,#6604,.T.);
#9163=ORIENTED_EDGE('',*,*,#6605,.T.);
#9164=ORIENTED_EDGE('',*,*,#6456,.F.);
#9165=ORIENTED_EDGE('',*,*,#6607,.T.);
#9166=ORIENTED_EDGE('',*,*,#6416,.T.);
#9167=ORIENTED_EDGE('',*,*,#6613,.T.);
#9168=ORIENTED_EDGE('',*,*,#6615,.T.);
#9169=ORIENTED_EDGE('',*,*,#6616,.T.);
#9170=ORIENTED_EDGE('',*,*,#6452,.F.);
#9171=ORIENTED_EDGE('',*,*,#6618,.T.);
#9172=ORIENTED_EDGE('',*,*,#6414,.T.);
#9173=ORIENTED_EDGE('',*,*,#6624,.T.);
#9174=ORIENTED_EDGE('',*,*,#6626,.T.);
#9175=ORIENTED_EDGE('',*,*,#6627,.T.);
#9176=ORIENTED_EDGE('',*,*,#6448,.F.);
#9177=ORIENTED_EDGE('',*,*,#6629,.T.);
#9178=ORIENTED_EDGE('',*,*,#6412,.T.);
#9179=ORIENTED_EDGE('',*,*,#6635,.T.);
#9180=ORIENTED_EDGE('',*,*,#6637,.T.);
#9181=ORIENTED_EDGE('',*,*,#6638,.T.);
#9182=ORIENTED_EDGE('',*,*,#6444,.F.);
#9183=ORIENTED_EDGE('',*,*,#6640,.T.);
#9184=ORIENTED_EDGE('',*,*,#6410,.T.);
#9185=ORIENTED_EDGE('',*,*,#6646,.T.);
#9186=ORIENTED_EDGE('',*,*,#6648,.T.);
#9187=ORIENTED_EDGE('',*,*,#6649,.T.);
#9188=ORIENTED_EDGE('',*,*,#6433,.F.);
#9189=ORIENTED_EDGE('',*,*,#6651,.T.);
#9190=ORIENTED_EDGE('',*,*,#6408,.T.);
#9191=ORIENTED_EDGE('',*,*,#6428,.T.);
#9192=ORIENTED_EDGE('',*,*,#6657,.T.);
#9193=ORIENTED_EDGE('',*,*,#6659,.T.);
#9194=ORIENTED_EDGE('',*,*,#6660,.T.);
#9195=ORIENTED_EDGE('',*,*,#6436,.F.);
#9196=ORIENTED_EDGE('',*,*,#6464,.F.);
#9197=ORIENTED_EDGE('',*,*,#6662,.T.);
#9198=ORIENTED_EDGE('',*,*,#6426,.T.);
#9199=ORIENTED_EDGE('',*,*,#6668,.T.);
#9200=ORIENTED_EDGE('',*,*,#6670,.T.);
#9201=ORIENTED_EDGE('',*,*,#6671,.T.);
#9202=ORIENTED_EDGE('',*,*,#6435,.T.);
#9203=ORIENTED_EDGE('',*,*,#6406,.F.);
#9204=ORIENTED_EDGE('',*,*,#6558,.T.);
#9205=ORIENTED_EDGE('',*,*,#6674,.T.);
#9206=ORIENTED_EDGE('',*,*,#6561,.T.);
#9207=ORIENTED_EDGE('',*,*,#6403,.F.);
#9208=ORIENTED_EDGE('',*,*,#6560,.T.);
#9209=ORIENTED_EDGE('',*,*,#6675,.T.);
#9210=ORIENTED_EDGE('',*,*,#6562,.T.);
#9211=ORIENTED_EDGE('',*,*,#6674,.F.);
#9212=ORIENTED_EDGE('',*,*,#6559,.T.);
#9213=ORIENTED_EDGE('',*,*,#6405,.T.);
#9214=ORIENTED_EDGE('',*,*,#6563,.T.);
#9215=ORIENTED_EDGE('',*,*,#6675,.F.);
#11015=CYLINDRICAL_SURFACE('',#12437,9.5);
#11016=CYLINDRICAL_SURFACE('',#12440,120.);
#11017=CYLINDRICAL_SURFACE('',#12463,160.);
#11018=CYLINDRICAL_SURFACE('',#12488,35.);
#11019=CYLINDRICAL_SURFACE('',#12489,30.);
#11020=CYLINDRICAL_SURFACE('',#12518,156.);
#11021=CYLINDRICAL_SURFACE('',#12523,10.);
#11022=CYLINDRICAL_SURFACE('',#12527,156.);
#11023=CYLINDRICAL_SURFACE('',#12535,156.);
#11024=CYLINDRICAL_SURFACE('',#12543,156.);
#11025=CYLINDRICAL_SURFACE('',#12551,156.);
#11026=CYLINDRICAL_SURFACE('',#12559,156.);
#11027=CYLINDRICAL_SURFACE('',#12567,156.);
#11028=CYLINDRICAL_SURFACE('',#12575,156.);
#11029=CYLINDRICAL_SURFACE('',#12583,156.);
#11030=CYLINDRICAL_SURFACE('',#12591,156.);
#11031=CYLINDRICAL_SURFACE('',#12596,10.);
#11032=CYLINDRICAL_SURFACE('',#12597,9.99999999999999);
#11033=CYLINDRICAL_SURFACE('',#12598,10.);
#11034=CYLINDRICAL_SURFACE('',#12599,10.);
#11035=CYLINDRICAL_SURFACE('',#12600,10.);
#11036=CYLINDRICAL_SURFACE('',#12601,10.);
#11037=CYLINDRICAL_SURFACE('',#12602,10.);
#11038=CYLINDRICAL_SURFACE('',#12603,10.);
#11039=CYLINDRICAL_SURFACE('',#12604,10.);
#11391=ADVANCED_FACE('',(#952),#625,.T.);
#11392=ADVANCED_FACE('',(#953),#626,.T.);
#11393=ADVANCED_FACE('',(#954),#627,.T.);
#11394=ADVANCED_FACE('',(#955),#11015,.F.);
#11395=ADVANCED_FACE('',(#956),#11016,.F.);
#11396=ADVANCED_FACE('',(#957,#569,#570,#571,#572,#573,#574,#575,#576,#577),
#11017,.T.);
#11397=ADVANCED_FACE('',(#958),#11018,.T.);
#11398=ADVANCED_FACE('',(#959),#11019,.T.);
#11399=ADVANCED_FACE('',(#960),#248,.T.);
#11400=ADVANCED_FACE('',(#961),#249,.T.);
#11401=ADVANCED_FACE('',(#962),#250,.T.);
#11402=ADVANCED_FACE('',(#963),#251,.T.);
#11403=ADVANCED_FACE('',(#964),#252,.T.);
#11404=ADVANCED_FACE('',(#965),#253,.T.);
#11405=ADVANCED_FACE('',(#966),#254,.T.);
#11406=ADVANCED_FACE('',(#967),#255,.T.);
#11407=ADVANCED_FACE('',(#968),#256,.T.);
#11408=ADVANCED_FACE('',(#969),#257,.T.);
#11409=ADVANCED_FACE('',(#970,#578),#258,.T.);
#11410=ADVANCED_FACE('',(#971,#579),#259,.F.);
#11411=ADVANCED_FACE('',(#972,#580),#260,.F.);
#11412=ADVANCED_FACE('',(#973,#581),#261,.F.);
#11413=ADVANCED_FACE('',(#974),#262,.F.);
#11414=ADVANCED_FACE('',(#975),#263,.F.);
#11415=ADVANCED_FACE('',(#976),#11020,.F.);
#11416=ADVANCED_FACE('',(#977),#264,.F.);
#11417=ADVANCED_FACE('',(#978),#265,.F.);
#11418=ADVANCED_FACE('',(#979),#11021,.T.);
#11419=ADVANCED_FACE('',(#980),#266,.F.);
#11420=ADVANCED_FACE('',(#981),#267,.F.);
#11421=ADVANCED_FACE('',(#982),#11022,.F.);
#11422=ADVANCED_FACE('',(#983),#268,.F.);
#11423=ADVANCED_FACE('',(#984),#269,.F.);
#11424=ADVANCED_FACE('',(#985),#270,.F.);
#11425=ADVANCED_FACE('',(#986),#271,.F.);
#11426=ADVANCED_FACE('',(#987),#11023,.F.);
#11427=ADVANCED_FACE('',(#988),#272,.F.);
#11428=ADVANCED_FACE('',(#989),#273,.F.);
#11429=ADVANCED_FACE('',(#990),#274,.F.);
#11430=ADVANCED_FACE('',(#991),#275,.F.);
#11431=ADVANCED_FACE('',(#992),#11024,.F.);
#11432=ADVANCED_FACE('',(#993),#276,.F.);
#11433=ADVANCED_FACE('',(#994),#277,.F.);
#11434=ADVANCED_FACE('',(#995),#278,.F.);
#11435=ADVANCED_FACE('',(#996),#279,.F.);
#11436=ADVANCED_FACE('',(#997),#11025,.F.);
#11437=ADVANCED_FACE('',(#998),#280,.F.);
#11438=ADVANCED_FACE('',(#999),#281,.F.);
#11439=ADVANCED_FACE('',(#1000),#282,.F.);
#11440=ADVANCED_FACE('',(#1001),#283,.F.);
#11441=ADVANCED_FACE('',(#1002),#11026,.F.);
#11442=ADVANCED_FACE('',(#1003),#284,.F.);
#11443=ADVANCED_FACE('',(#1004),#285,.F.);
#11444=ADVANCED_FACE('',(#1005),#286,.F.);
#11445=ADVANCED_FACE('',(#1006),#287,.F.);
#11446=ADVANCED_FACE('',(#1007),#11027,.F.);
#11447=ADVANCED_FACE('',(#1008),#288,.F.);
#11448=ADVANCED_FACE('',(#1009),#289,.F.);
#11449=ADVANCED_FACE('',(#1010),#290,.F.);
#11450=ADVANCED_FACE('',(#1011),#291,.F.);
#11451=ADVANCED_FACE('',(#1012),#11028,.F.);
#11452=ADVANCED_FACE('',(#1013),#292,.F.);
#11453=ADVANCED_FACE('',(#1014),#293,.F.);
#11454=ADVANCED_FACE('',(#1015),#294,.F.);
#11455=ADVANCED_FACE('',(#1016),#295,.F.);
#11456=ADVANCED_FACE('',(#1017),#11029,.F.);
#11457=ADVANCED_FACE('',(#1018),#296,.F.);
#11458=ADVANCED_FACE('',(#1019),#297,.F.);
#11459=ADVANCED_FACE('',(#1020),#298,.F.);
#11460=ADVANCED_FACE('',(#1021),#299,.F.);
#11461=ADVANCED_FACE('',(#1022),#11030,.F.);
#11462=ADVANCED_FACE('',(#1023),#300,.F.);
#11463=ADVANCED_FACE('',(#1024),#301,.F.);
#11464=ADVANCED_FACE('',(#1025),#11031,.T.);
#11465=ADVANCED_FACE('',(#1026),#11032,.T.);
#11466=ADVANCED_FACE('',(#1027),#11033,.T.);
#11467=ADVANCED_FACE('',(#1028),#11034,.T.);
#11468=ADVANCED_FACE('',(#1029),#11035,.T.);
#11469=ADVANCED_FACE('',(#1030),#11036,.T.);
#11470=ADVANCED_FACE('',(#1031),#11037,.T.);
#11471=ADVANCED_FACE('',(#1032),#11038,.T.);
#11472=ADVANCED_FACE('',(#1033),#11039,.T.);
#11473=ADVANCED_FACE('',(#1034),#302,.F.);
#11474=ADVANCED_FACE('',(#1035),#303,.F.);
#11475=ADVANCED_FACE('',(#1036),#304,.F.);
#11476=ADVANCED_FACE('',(#1037),#305,.F.);
#11477=ADVANCED_FACE('',(#1038),#306,.F.);
#11478=ADVANCED_FACE('',(#1039),#307,.F.);
#11479=ADVANCED_FACE('',(#1040),#308,.F.);
#11480=ADVANCED_FACE('',(#1041),#309,.F.);
#11481=ADVANCED_FACE('',(#1042),#310,.F.);
#11482=ADVANCED_FACE('',(#1043),#311,.F.);
#11483=ADVANCED_FACE('',(#1044,#582),#312,.T.);
#11484=ADVANCED_FACE('',(#1045),#313,.F.);
#11485=ADVANCED_FACE('',(#1046),#314,.F.);
#11486=ADVANCED_FACE('',(#1047),#315,.F.);
#11824=CLOSED_SHELL('',(#11391,#11392,#11393,#11394,#11395,#11396,#11397,
#11398,#11399,#11400,#11401,#11402,#11403,#11404,#11405,#11406,#11407,#11408,
#11409,#11410,#11411,#11412,#11413,#11414,#11415,#11416,#11417,#11418,#11419,
#11420,#11421,#11422,#11423,#11424,#11425,#11426,#11427,#11428,#11429,#11430,
#11431,#11432,#11433,#11434,#11435,#11436,#11437,#11438,#11439,#11440,#11441,
#11442,#11443,#11444,#11445,#11446,#11447,#11448,#11449,#11450,#11451,#11452,
#11453,#11454,#11455,#11456,#11457,#11458,#11459,#11460,#11461,#11462,#11463,
#11464,#11465,#11466,#11467,#11468,#11469,#11470,#11471,#11472,#11473,#11474,
#11475,#11476,#11477,#11478,#11479,#11480,#11481,#11482,#11483,#11484,#11485,
#11486));
#12424=AXIS2_PLACEMENT_3D('',#25203,#14423,#14424);
#12425=AXIS2_PLACEMENT_3D('',#25204,#14425,#14426);
#12426=AXIS2_PLACEMENT_3D('',#25206,#14427,#14428);
#12427=AXIS2_PLACEMENT_3D('',#25210,#14430,#14431);
#12428=AXIS2_PLACEMENT_3D('',#25211,#14432,#14433);
#12429=AXIS2_PLACEMENT_3D('',#25212,#14434,#14435);
#12430=AXIS2_PLACEMENT_3D('',#25215,#14436,#14437);
#12431=AXIS2_PLACEMENT_3D('',#25216,#14438,#14439);
#12432=AXIS2_PLACEMENT_3D('',#25219,#14441,#14442);
#12433=AXIS2_PLACEMENT_3D('',#25220,#14443,#14444);
#12434=AXIS2_PLACEMENT_3D('',#25223,#14445,#14446);
#12435=AXIS2_PLACEMENT_3D('',#25224,#14447,#14448);
#12436=AXIS2_PLACEMENT_3D('',#25227,#14450,#14451);
#12437=AXIS2_PLACEMENT_3D('',#25228,#14452,#14453);
#12438=AXIS2_PLACEMENT_3D('',#25231,#14454,#14455);
#12439=AXIS2_PLACEMENT_3D('',#25235,#14457,#14458);
#12440=AXIS2_PLACEMENT_3D('',#25237,#14460,#14461);
#12441=AXIS2_PLACEMENT_3D('',#25239,#14462,#14463);
#12442=AXIS2_PLACEMENT_3D('',#25243,#14465,#14466);
#12443=AXIS2_PLACEMENT_3D('',#25245,#14467,#14468);
#12444=AXIS2_PLACEMENT_3D('',#25247,#14469,#14470);
#12445=AXIS2_PLACEMENT_3D('',#25249,#14471,#14472);
#12446=AXIS2_PLACEMENT_3D('',#25251,#14473,#14474);
#12447=AXIS2_PLACEMENT_3D('',#25253,#14475,#14476);
#12448=AXIS2_PLACEMENT_3D('',#25255,#14477,#14478);
#12449=AXIS2_PLACEMENT_3D('',#25257,#14479,#14480);
#12450=AXIS2_PLACEMENT_3D('',#25259,#14481,#14482);
#12451=AXIS2_PLACEMENT_3D('',#25261,#14483,#14484);
#12452=AXIS2_PLACEMENT_3D('',#25263,#14485,#14486);
#12453=AXIS2_PLACEMENT_3D('',#25265,#14487,#14488);
#12454=AXIS2_PLACEMENT_3D('',#25267,#14489,#14490);
#12455=AXIS2_PLACEMENT_3D('',#25269,#14491,#14492);
#12456=AXIS2_PLACEMENT_3D('',#25271,#14493,#14494);
#12457=AXIS2_PLACEMENT_3D('',#25273,#14495,#14496);
#12458=AXIS2_PLACEMENT_3D('',#25275,#14497,#14498);
#12459=AXIS2_PLACEMENT_3D('',#25277,#14499,#14500);
#12460=AXIS2_PLACEMENT_3D('',#25279,#14501,#14502);
#12461=AXIS2_PLACEMENT_3D('',#25281,#14503,#14504);
#12462=AXIS2_PLACEMENT_3D('',#25282,#14505,#14506);
#12463=AXIS2_PLACEMENT_3D('',#25283,#14507,#14508);
#12464=AXIS2_PLACEMENT_3D('',#25285,#14509,#14510);
#12465=AXIS2_PLACEMENT_3D('',#25289,#14512,#14513);
#12466=AXIS2_PLACEMENT_3D('',#25293,#14515,#14516);
#12467=AXIS2_PLACEMENT_3D('',#25296,#14518,#14519);
#12468=AXIS2_PLACEMENT_3D('',#25298,#14520,#14521);
#12469=AXIS2_PLACEMENT_3D('',#25301,#14523,#14524);
#12470=AXIS2_PLACEMENT_3D('',#25304,#14525,#14526);
#12471=AXIS2_PLACEMENT_3D('',#25308,#14528,#14529);
#12472=AXIS2_PLACEMENT_3D('',#25314,#14532,#14533);
#12473=AXIS2_PLACEMENT_3D('',#25317,#14535,#14536);
#12474=AXIS2_PLACEMENT_3D('',#25322,#14538,#14539);
#12475=AXIS2_PLACEMENT_3D('',#25325,#14541,#14542);
#12476=AXIS2_PLACEMENT_3D('',#25330,#14544,#14545);
#12477=AXIS2_PLACEMENT_3D('',#25333,#14547,#14548);
#12478=AXIS2_PLACEMENT_3D('',#25338,#14550,#14551);
#12479=AXIS2_PLACEMENT_3D('',#25341,#14553,#14554);
#12480=AXIS2_PLACEMENT_3D('',#25344,#14555,#14556);
#12481=AXIS2_PLACEMENT_3D('',#25348,#14558,#14559);
#12482=AXIS2_PLACEMENT_3D('',#25354,#14562,#14563);
#12483=AXIS2_PLACEMENT_3D('',#25357,#14565,#14566);
#12484=AXIS2_PLACEMENT_3D('',#25362,#14568,#14569);
#12485=AXIS2_PLACEMENT_3D('',#25365,#14571,#14572);
#12486=AXIS2_PLACEMENT_3D('',#25370,#14574,#14575);
#12487=AXIS2_PLACEMENT_3D('',#25373,#14577,#14578);
#12488=AXIS2_PLACEMENT_3D('',#25374,#14579,#14580);
#12489=AXIS2_PLACEMENT_3D('',#25376,#14582,#14583);
#12490=AXIS2_PLACEMENT_3D('',#25379,#14585,#14586);
#12491=AXIS2_PLACEMENT_3D('',#25380,#14587,#14588);
#12492=AXIS2_PLACEMENT_3D('',#25386,#14592,#14593);
#12493=AXIS2_PLACEMENT_3D('',#25392,#14597,#14598);
#12494=AXIS2_PLACEMENT_3D('',#25398,#14602,#14603);
#12495=AXIS2_PLACEMENT_3D('',#25404,#14607,#14608);
#12496=AXIS2_PLACEMENT_3D('',#25410,#14612,#14613);
#12497=AXIS2_PLACEMENT_3D('',#25416,#14617,#14618);
#12498=AXIS2_PLACEMENT_3D('',#25422,#14622,#14623);
#12499=AXIS2_PLACEMENT_3D('',#25428,#14627,#14628);
#12500=AXIS2_PLACEMENT_3D('',#25434,#14632,#14633);
#12501=AXIS2_PLACEMENT_3D('',#25440,#14637,#14638);
#12502=AXIS2_PLACEMENT_3D('',#25444,#14640,#14641);
#12503=AXIS2_PLACEMENT_3D('',#25453,#14646,#14647);
#12504=AXIS2_PLACEMENT_3D('',#25462,#14652,#14653);
#12505=AXIS2_PLACEMENT_3D('',#25471,#14658,#14659);
#12506=AXIS2_PLACEMENT_3D('',#25480,#14664,#14665);
#12507=AXIS2_PLACEMENT_3D('',#25489,#14670,#14671);
#12508=AXIS2_PLACEMENT_3D('',#25498,#14676,#14677);
#12509=AXIS2_PLACEMENT_3D('',#25507,#14682,#14683);
#12510=AXIS2_PLACEMENT_3D('',#25516,#14688,#14689);
#12511=AXIS2_PLACEMENT_3D('',#25525,#14694,#14695);
#12512=AXIS2_PLACEMENT_3D('',#25536,#14702,#14703);
#12513=AXIS2_PLACEMENT_3D('',#25542,#14707,#14708);
#12514=AXIS2_PLACEMENT_3D('',#25543,#14709,#14710);
#12515=AXIS2_PLACEMENT_3D('',#25544,#14711,#14712);
#12516=AXIS2_PLACEMENT_3D('',#25550,#14716,#14717);
#12517=AXIS2_PLACEMENT_3D('',#25551,#14718,#14719);
#12518=AXIS2_PLACEMENT_3D('',#25555,#14722,#14723);
#12519=AXIS2_PLACEMENT_3D('',#25558,#14725,#14726);
#12520=AXIS2_PLACEMENT_3D('',#25559,#14727,#14728);
#12521=AXIS2_PLACEMENT_3D('',#25561,#14730,#14731);
#12522=AXIS2_PLACEMENT_3D('',#25562,#14732,#14733);
#12523=AXIS2_PLACEMENT_3D('',#25564,#14735,#14736);
#12524=AXIS2_PLACEMENT_3D('',#25565,#14737,#14738);
#12525=AXIS2_PLACEMENT_3D('',#25571,#14742,#14743);
#12526=AXIS2_PLACEMENT_3D('',#25572,#14744,#14745);
#12527=AXIS2_PLACEMENT_3D('',#25576,#14748,#14749);
#12528=AXIS2_PLACEMENT_3D('',#25579,#14751,#14752);
#12529=AXIS2_PLACEMENT_3D('',#25580,#14753,#14754);
#12530=AXIS2_PLACEMENT_3D('',#25582,#14756,#14757);
#12531=AXIS2_PLACEMENT_3D('',#25583,#14758,#14759);
#12532=AXIS2_PLACEMENT_3D('',#25585,#14761,#14762);
#12533=AXIS2_PLACEMENT_3D('',#25591,#14766,#14767);
#12534=AXIS2_PLACEMENT_3D('',#25592,#14768,#14769);
#12535=AXIS2_PLACEMENT_3D('',#25596,#14772,#14773);
#12536=AXIS2_PLACEMENT_3D('',#25599,#14775,#14776);
#12537=AXIS2_PLACEMENT_3D('',#25600,#14777,#14778);
#12538=AXIS2_PLACEMENT_3D('',#25602,#14780,#14781);
#12539=AXIS2_PLACEMENT_3D('',#25603,#14782,#14783);
#12540=AXIS2_PLACEMENT_3D('',#25605,#14785,#14786);
#12541=AXIS2_PLACEMENT_3D('',#25611,#14790,#14791);
#12542=AXIS2_PLACEMENT_3D('',#25612,#14792,#14793);
#12543=AXIS2_PLACEMENT_3D('',#25616,#14796,#14797);
#12544=AXIS2_PLACEMENT_3D('',#25619,#14799,#14800);
#12545=AXIS2_PLACEMENT_3D('',#25620,#14801,#14802);
#12546=AXIS2_PLACEMENT_3D('',#25622,#14804,#14805);
#12547=AXIS2_PLACEMENT_3D('',#25623,#14806,#14807);
#12548=AXIS2_PLACEMENT_3D('',#25625,#14809,#14810);
#12549=AXIS2_PLACEMENT_3D('',#25631,#14814,#14815);
#12550=AXIS2_PLACEMENT_3D('',#25632,#14816,#14817);
#12551=AXIS2_PLACEMENT_3D('',#25636,#14820,#14821);
#12552=AXIS2_PLACEMENT_3D('',#25639,#14823,#14824);
#12553=AXIS2_PLACEMENT_3D('',#25640,#14825,#14826);
#12554=AXIS2_PLACEMENT_3D('',#25642,#14828,#14829);
#12555=AXIS2_PLACEMENT_3D('',#25643,#14830,#14831);
#12556=AXIS2_PLACEMENT_3D('',#25645,#14833,#14834);
#12557=AXIS2_PLACEMENT_3D('',#25651,#14838,#14839);
#12558=AXIS2_PLACEMENT_3D('',#25652,#14840,#14841);
#12559=AXIS2_PLACEMENT_3D('',#25656,#14844,#14845);
#12560=AXIS2_PLACEMENT_3D('',#25659,#14847,#14848);
#12561=AXIS2_PLACEMENT_3D('',#25660,#14849,#14850);
#12562=AXIS2_PLACEMENT_3D('',#25662,#14852,#14853);
#12563=AXIS2_PLACEMENT_3D('',#25663,#14854,#14855);
#12564=AXIS2_PLACEMENT_3D('',#25665,#14857,#14858);
#12565=AXIS2_PLACEMENT_3D('',#25671,#14862,#14863);
#12566=AXIS2_PLACEMENT_3D('',#25672,#14864,#14865);
#12567=AXIS2_PLACEMENT_3D('',#25676,#14868,#14869);
#12568=AXIS2_PLACEMENT_3D('',#25679,#14871,#14872);
#12569=AXIS2_PLACEMENT_3D('',#25680,#14873,#14874);
#12570=AXIS2_PLACEMENT_3D('',#25682,#14876,#14877);
#12571=AXIS2_PLACEMENT_3D('',#25683,#14878,#14879);
#12572=AXIS2_PLACEMENT_3D('',#25685,#14881,#14882);
#12573=AXIS2_PLACEMENT_3D('',#25691,#14886,#14887);
#12574=AXIS2_PLACEMENT_3D('',#25692,#14888,#14889);
#12575=AXIS2_PLACEMENT_3D('',#25696,#14892,#14893);
#12576=AXIS2_PLACEMENT_3D('',#25699,#14895,#14896);
#12577=AXIS2_PLACEMENT_3D('',#25700,#14897,#14898);
#12578=AXIS2_PLACEMENT_3D('',#25702,#14900,#14901);
#12579=AXIS2_PLACEMENT_3D('',#25703,#14902,#14903);
#12580=AXIS2_PLACEMENT_3D('',#25705,#14905,#14906);
#12581=AXIS2_PLACEMENT_3D('',#25711,#14910,#14911);
#12582=AXIS2_PLACEMENT_3D('',#25712,#14912,#14913);
#12583=AXIS2_PLACEMENT_3D('',#25716,#14916,#14917);
#12584=AXIS2_PLACEMENT_3D('',#25719,#14919,#14920);
#12585=AXIS2_PLACEMENT_3D('',#25720,#14921,#14922);
#12586=AXIS2_PLACEMENT_3D('',#25722,#14924,#14925);
#12587=AXIS2_PLACEMENT_3D('',#25723,#14926,#14927);
#12588=AXIS2_PLACEMENT_3D('',#25725,#14929,#14930);
#12589=AXIS2_PLACEMENT_3D('',#25731,#14934,#14935);
#12590=AXIS2_PLACEMENT_3D('',#25732,#14936,#14937);
#12591=AXIS2_PLACEMENT_3D('',#25736,#14940,#14941);
#12592=AXIS2_PLACEMENT_3D('',#25739,#14943,#14944);
#12593=AXIS2_PLACEMENT_3D('',#25740,#14945,#14946);
#12594=AXIS2_PLACEMENT_3D('',#25742,#14948,#14949);
#12595=AXIS2_PLACEMENT_3D('',#25743,#14950,#14951);
#12596=AXIS2_PLACEMENT_3D('',#25745,#14953,#14954);
#12597=AXIS2_PLACEMENT_3D('',#25746,#14955,#14956);
#12598=AXIS2_PLACEMENT_3D('',#25747,#14957,#14958);
#12599=AXIS2_PLACEMENT_3D('',#25748,#14959,#14960);
#12600=AXIS2_PLACEMENT_3D('',#25749,#14961,#14962);
#12601=AXIS2_PLACEMENT_3D('',#25750,#14963,#14964);
#12602=AXIS2_PLACEMENT_3D('',#25751,#14965,#14966);
#12603=AXIS2_PLACEMENT_3D('',#25752,#14967,#14968);
#12604=AXIS2_PLACEMENT_3D('',#25753,#14969,#14970);
#12605=AXIS2_PLACEMENT_3D('',#25754,#14971,#14972);
#12606=AXIS2_PLACEMENT_3D('',#25755,#14973,#14974);
#12607=AXIS2_PLACEMENT_3D('',#25756,#14975,#14976);
#12608=AXIS2_PLACEMENT_3D('',#25757,#14977,#14978);
#12609=AXIS2_PLACEMENT_3D('',#25758,#14979,#14980);
#12610=AXIS2_PLACEMENT_3D('',#25759,#14981,#14982);
#12611=AXIS2_PLACEMENT_3D('',#25760,#14983,#14984);
#12612=AXIS2_PLACEMENT_3D('',#25761,#14985,#14986);
#12613=AXIS2_PLACEMENT_3D('',#25762,#14987,#14988);
#12614=AXIS2_PLACEMENT_3D('',#25763,#14989,#14990);
#12615=AXIS2_PLACEMENT_3D('',#25764,#14991,#14992);
#12616=AXIS2_PLACEMENT_3D('',#25765,#14993,#14994);
#12617=AXIS2_PLACEMENT_3D('',#25767,#14996,#14997);
#12618=AXIS2_PLACEMENT_3D('',#25769,#14999,#15000);
#14423=DIRECTION('axis',(0.,0.,1.));
#14424=DIRECTION('refdir',(1.,0.,0.));
#14425=DIRECTION('center_axis',(0.,0.,1.));
#14426=DIRECTION('ref_axis',(1.,0.,0.));
#14427=DIRECTION('center_axis',(0.,0.,1.));
#14428=DIRECTION('ref_axis',(1.,0.,0.));
#14429=DIRECTION('',(0.707106781186541,8.65956056235485E-17,-0.707106781186554));
#14430=DIRECTION('center_axis',(0.,0.,-1.));
#14431=DIRECTION('ref_axis',(1.,0.,0.));
#14432=DIRECTION('center_axis',(0.,0.,-1.));
#14433=DIRECTION('ref_axis',(1.,0.,0.));
#14434=DIRECTION('center_axis',(0.,0.,1.));
#14435=DIRECTION('ref_axis',(1.,0.,0.));
#14436=DIRECTION('center_axis',(0.,0.,1.));
#14437=DIRECTION('ref_axis',(1.,0.,0.));
#14438=DIRECTION('center_axis',(0.,0.,1.));
#14439=DIRECTION('ref_axis',(1.,0.,0.));
#14440=DIRECTION('',(0.707106781186529,8.65956056235471E-17,-0.707106781186566));
#14441=DIRECTION('center_axis',(0.,0.,-1.));
#14442=DIRECTION('ref_axis',(1.,0.,0.));
#14443=DIRECTION('center_axis',(0.,0.,1.));
#14444=DIRECTION('ref_axis',(1.,0.,0.));
#14445=DIRECTION('center_axis',(0.,0.,1.));
#14446=DIRECTION('ref_axis',(1.,0.,0.));
#14447=DIRECTION('center_axis',(0.,0.,1.));
#14448=DIRECTION('ref_axis',(1.,0.,0.));
#14449=DIRECTION('',(0.707106781186545,8.6595605623549E-17,-0.70710678118655));
#14450=DIRECTION('center_axis',(0.,0.,-1.));
#14451=DIRECTION('ref_axis',(1.,0.,0.));
#14452=DIRECTION('center_axis',(0.,0.,-1.));
#14453=DIRECTION('ref_axis',(1.83697019872103E-16,-1.,0.));
#14454=DIRECTION('center_axis',(0.,0.,1.));
#14455=DIRECTION('ref_axis',(1.,0.,0.));
#14456=DIRECTION('',(0.,0.,-1.));
#14457=DIRECTION('center_axis',(0.,0.,-1.));
#14458=DIRECTION('ref_axis',(-1.,0.,0.));
#14459=DIRECTION('',(0.,0.,-1.));
#14460=DIRECTION('center_axis',(0.,0.,-1.));
#14461=DIRECTION('ref_axis',(-1.,0.,0.));
#14462=DIRECTION('center_axis',(0.,0.,1.));
#14463=DIRECTION('ref_axis',(1.,0.,0.));
#14464=DIRECTION('',(0.,0.,-1.));
#14465=DIRECTION('center_axis',(0.,0.,1.));
#14466=DIRECTION('ref_axis',(1.,0.,0.));
#14467=DIRECTION('center_axis',(0.,0.,1.));
#14468=DIRECTION('ref_axis',(1.,0.,0.));
#14469=DIRECTION('center_axis',(0.,0.,1.));
#14470=DIRECTION('ref_axis',(1.,0.,0.));
#14471=DIRECTION('center_axis',(0.,0.,1.));
#14472=DIRECTION('ref_axis',(1.,0.,0.));
#14473=DIRECTION('center_axis',(0.,0.,1.));
#14474=DIRECTION('ref_axis',(1.,0.,0.));
#14475=DIRECTION('center_axis',(0.,0.,1.));
#14476=DIRECTION('ref_axis',(1.,0.,0.));
#14477=DIRECTION('center_axis',(0.,0.,1.));
#14478=DIRECTION('ref_axis',(1.,0.,0.));
#14479=DIRECTION('center_axis',(0.,0.,1.));
#14480=DIRECTION('ref_axis',(1.,0.,0.));
#14481=DIRECTION('center_axis',(0.,0.,1.));
#14482=DIRECTION('ref_axis',(1.,0.,0.));
#14483=DIRECTION('center_axis',(0.,0.,1.));
#14484=DIRECTION('ref_axis',(1.,0.,0.));
#14485=DIRECTION('center_axis',(0.,0.,1.));
#14486=DIRECTION('ref_axis',(1.,0.,0.));
#14487=DIRECTION('center_axis',(0.,0.,1.));
#14488=DIRECTION('ref_axis',(1.,0.,0.));
#14489=DIRECTION('center_axis',(0.,0.,1.));
#14490=DIRECTION('ref_axis',(1.,0.,0.));
#14491=DIRECTION('center_axis',(0.,0.,1.));
#14492=DIRECTION('ref_axis',(1.,0.,0.));
#14493=DIRECTION('center_axis',(0.,0.,1.));
#14494=DIRECTION('ref_axis',(1.,0.,0.));
#14495=DIRECTION('center_axis',(0.,0.,1.));
#14496=DIRECTION('ref_axis',(1.,0.,0.));
#14497=DIRECTION('center_axis',(0.,0.,1.));
#14498=DIRECTION('ref_axis',(1.,0.,0.));
#14499=DIRECTION('center_axis',(0.,0.,-1.));
#14500=DIRECTION('ref_axis',(1.,-3.5527136788005E-14,0.));
#14501=DIRECTION('center_axis',(0.,0.,1.));
#14502=DIRECTION('ref_axis',(1.,0.,0.));
#14503=DIRECTION('center_axis',(0.,0.,1.));
#14504=DIRECTION('ref_axis',(1.,0.,0.));
#14505=DIRECTION('center_axis',(0.,0.,1.));
#14506=DIRECTION('ref_axis',(1.,0.,0.));
#14507=DIRECTION('center_axis',(0.,0.,-1.));
#14508=DIRECTION('ref_axis',(-1.,0.,0.));
#14509=DIRECTION('center_axis',(0.,0.,1.));
#14510=DIRECTION('ref_axis',(1.,0.,0.));
#14511=DIRECTION('',(0.,0.,1.));
#14512=DIRECTION('center_axis',(0.,0.,1.));
#14513=DIRECTION('ref_axis',(1.,0.,0.));
#14514=DIRECTION('',(0.,0.,-1.));
#14515=DIRECTION('center_axis',(0.,0.,1.));
#14516=DIRECTION('ref_axis',(1.,0.,0.));
#14517=DIRECTION('',(0.,0.,1.));
#14518=DIRECTION('center_axis',(0.,0.,1.));
#14519=DIRECTION('ref_axis',(1.,0.,0.));
#14520=DIRECTION('center_axis',(0.,0.,1.));
#14521=DIRECTION('ref_axis',(1.,0.,0.));
#14522=DIRECTION('',(0.,0.,-1.));
#14523=DIRECTION('center_axis',(0.,0.,1.));
#14524=DIRECTION('ref_axis',(1.,0.,0.));
#14525=DIRECTION('center_axis',(0.,0.,1.));
#14526=DIRECTION('ref_axis',(1.,0.,0.));
#14527=DIRECTION('',(0.,0.,-1.));
#14528=DIRECTION('center_axis',(0.,0.,1.));
#14529=DIRECTION('ref_axis',(1.,0.,0.));
#14530=DIRECTION('',(0.,0.,-1.));
#14531=DIRECTION('',(0.,0.,-1.));
#14532=DIRECTION('center_axis',(0.,0.,1.));
#14533=DIRECTION('ref_axis',(1.,0.,0.));
#14534=DIRECTION('',(0.,0.,-1.));
#14535=DIRECTION('center_axis',(0.,0.,1.));
#14536=DIRECTION('ref_axis',(1.,0.,0.));
#14537=DIRECTION('',(0.,0.,-1.));
#14538=DIRECTION('center_axis',(0.,0.,1.));
#14539=DIRECTION('ref_axis',(1.,0.,0.));
#14540=DIRECTION('',(0.,0.,-1.));
#14541=DIRECTION('center_axis',(0.,0.,1.));
#14542=DIRECTION('ref_axis',(1.,0.,0.));
#14543=DIRECTION('',(0.,0.,-1.));
#14544=DIRECTION('center_axis',(0.,0.,1.));
#14545=DIRECTION('ref_axis',(1.,0.,0.));
#14546=DIRECTION('',(0.,0.,-1.));
#14547=DIRECTION('center_axis',(0.,0.,1.));
#14548=DIRECTION('ref_axis',(1.,0.,0.));
#14549=DIRECTION('',(0.,0.,-1.));
#14550=DIRECTION('center_axis',(0.,0.,1.));
#14551=DIRECTION('ref_axis',(1.,0.,0.));
#14552=DIRECTION('',(0.,0.,-1.));
#14553=DIRECTION('center_axis',(0.,0.,1.));
#14554=DIRECTION('ref_axis',(1.,0.,0.));
#14555=DIRECTION('center_axis',(0.,0.,1.));
#14556=DIRECTION('ref_axis',(1.,0.,0.));
#14557=DIRECTION('',(0.,0.,-1.));
#14558=DIRECTION('center_axis',(0.,0.,1.));
#14559=DIRECTION('ref_axis',(1.,0.,0.));
#14560=DIRECTION('',(0.,0.,-1.));
#14561=DIRECTION('',(0.,0.,-1.));
#14562=DIRECTION('center_axis',(0.,0.,1.));
#14563=DIRECTION('ref_axis',(1.,0.,0.));
#14564=DIRECTION('',(0.,0.,-1.));
#14565=DIRECTION('center_axis',(0.,0.,1.));
#14566=DIRECTION('ref_axis',(1.,0.,0.));
#14567=DIRECTION('',(0.,0.,-1.));
#14568=DIRECTION('center_axis',(0.,0.,1.));
#14569=DIRECTION('ref_axis',(1.,0.,0.));
#14570=DIRECTION('',(0.,0.,-1.));
#14571=DIRECTION('center_axis',(0.,0.,1.));
#14572=DIRECTION('ref_axis',(1.,0.,0.));
#14573=DIRECTION('',(0.,0.,-1.));
#14574=DIRECTION('center_axis',(0.,0.,1.));
#14575=DIRECTION('ref_axis',(1.,0.,0.));
#14576=DIRECTION('',(0.,0.,-1.));
#14577=DIRECTION('center_axis',(0.,0.,1.));
#14578=DIRECTION('ref_axis',(1.,0.,0.));
#14579=DIRECTION('center_axis',(0.,0.,-1.));
#14580=DIRECTION('ref_axis',(-1.,0.,0.));
#14581=DIRECTION('',(0.,0.,1.));
#14582=DIRECTION('center_axis',(0.,0.,-1.));
#14583=DIRECTION('ref_axis',(-1.,0.,0.));
#14584=DIRECTION('',(0.,0.,1.));
#14585=DIRECTION('center_axis',(0.,0.,1.));
#14586=DIRECTION('ref_axis',(1.,0.,0.));
#14587=DIRECTION('center_axis',(0.,0.,1.));
#14588=DIRECTION('ref_axis',(1.,0.,0.));
#14589=DIRECTION('',(0.,-1.,0.));
#14590=DIRECTION('',(1.,0.,0.));
#14591=DIRECTION('',(0.,1.,0.));
#14592=DIRECTION('center_axis',(0.,0.,1.));
#14593=DIRECTION('ref_axis',(0.809016994374947,0.587785252292474,0.));
#14594=DIRECTION('',(0.587785252292474,-0.809016994374947,0.));
#14595=DIRECTION('',(0.809016994374947,0.587785252292474,0.));
#14596=DIRECTION('',(-0.587785252292474,0.809016994374947,0.));
#14597=DIRECTION('center_axis',(0.,0.,1.));
#14598=DIRECTION('ref_axis',(0.309016994374945,0.951056516295155,0.));
#14599=DIRECTION('',(0.951056516295154,-0.309016994374945,0.));
#14600=DIRECTION('',(0.309016994374945,0.951056516295154,0.));
#14601=DIRECTION('',(-0.951056516295154,0.309016994374945,0.));
#14602=DIRECTION('center_axis',(0.,0.,1.));
#14603=DIRECTION('ref_axis',(-0.309016994374952,0.951056516295152,0.));
#14604=DIRECTION('',(0.951056516295152,0.309016994374952,0.));
#14605=DIRECTION('',(-0.309016994374952,0.951056516295152,0.));
#14606=DIRECTION('',(-0.951056516295152,-0.309016994374952,0.));
#14607=DIRECTION('center_axis',(0.,0.,1.));
#14608=DIRECTION('ref_axis',(-0.809016994374951,0.587785252292469,0.));
#14609=DIRECTION('',(0.587785252292469,0.809016994374951,0.));
#14610=DIRECTION('',(-0.809016994374951,0.587785252292468,0.));
#14611=DIRECTION('',(-0.587785252292468,-0.809016994374951,0.));
#14612=DIRECTION('center_axis',(0.,0.,1.));
#14613=DIRECTION('ref_axis',(-1.,0.,0.));
#14614=DIRECTION('',(0.,1.,0.));
#14615=DIRECTION('',(-1.,0.,0.));
#14616=DIRECTION('',(0.,-1.,0.));
#14617=DIRECTION('center_axis',(0.,0.,1.));
#14618=DIRECTION('ref_axis',(-0.809016994374942,-0.58778525229248,0.));
#14619=DIRECTION('',(-0.58778525229248,0.809016994374942,0.));
#14620=DIRECTION('',(-0.809016994374942,-0.58778525229248,0.));
#14621=DIRECTION('',(0.58778525229248,-0.809016994374942,0.));
#14622=DIRECTION('center_axis',(0.,0.,1.));
#14623=DIRECTION('ref_axis',(-0.309016994374938,-0.951056516295157,0.));
#14624=DIRECTION('',(-0.951056516295157,0.309016994374938,0.));
#14625=DIRECTION('',(-0.309016994374938,-0.951056516295157,0.));
#14626=DIRECTION('',(0.951056516295157,-0.309016994374938,0.));
#14627=DIRECTION('center_axis',(0.,0.,1.));
#14628=DIRECTION('ref_axis',(0.309016994374958,-0.95105651629515,0.));
#14629=DIRECTION('',(-0.95105651629515,-0.309016994374958,0.));
#14630=DIRECTION('',(0.309016994374958,-0.95105651629515,0.));
#14631=DIRECTION('',(0.95105651629515,0.309016994374958,0.));
#14632=DIRECTION('center_axis',(0.,0.,1.));
#14633=DIRECTION('ref_axis',(0.809016994374955,-0.587785252292463,0.));
#14634=DIRECTION('',(-0.587785252292463,-0.809016994374955,0.));
#14635=DIRECTION('',(0.809016994374955,-0.587785252292463,0.));
#14636=DIRECTION('',(0.587785252292462,0.809016994374955,0.));
#14637=DIRECTION('center_axis',(0.,0.,1.));
#14638=DIRECTION('ref_axis',(1.,0.,0.));
#14639=DIRECTION('',(0.777145961456963,0.629320391049847,0.));
#14640=DIRECTION('center_axis',(0.,0.,-1.));
#14641=DIRECTION('ref_axis',(0.809016994374955,-0.587785252292462,0.));
#14642=DIRECTION('',(0.587785252292462,0.809016994374955,0.));
#14643=DIRECTION('',(0.809016994374955,-0.587785252292463,0.));
#14644=DIRECTION('',(-0.587785252292463,-0.809016994374955,0.));
#14645=DIRECTION('',(0.258819045102522,0.965925826289068,0.));
#14646=DIRECTION('center_axis',(0.,0.,-1.));
#14647=DIRECTION('ref_axis',(1.,0.,0.));
#14648=DIRECTION('',(0.,1.,0.));
#14649=DIRECTION('',(1.,0.,0.));
#14650=DIRECTION('',(0.,-1.,0.));
#14651=DIRECTION('',(-0.3583679495453,0.933580426497202,0.));
#14652=DIRECTION('center_axis',(0.,0.,-1.));
#14653=DIRECTION('ref_axis',(0.809016994374947,0.587785252292474,0.));
#14654=DIRECTION('',(-0.587785252292474,0.809016994374947,0.));
#14655=DIRECTION('',(0.809016994374947,0.587785252292474,0.));
#14656=DIRECTION('',(0.587785252292474,-0.809016994374947,0.));
#14657=DIRECTION('',(-0.838670567945425,0.544639035015026,0.));
#14658=DIRECTION('center_axis',(0.,0.,-1.));
#14659=DIRECTION('ref_axis',(0.309016994374945,0.951056516295154,0.));
#14660=DIRECTION('',(-0.951056516295154,0.309016994374945,0.));
#14661=DIRECTION('',(0.309016994374945,0.951056516295155,0.));
#14662=DIRECTION('',(0.951056516295154,-0.309016994374945,0.));
#14663=DIRECTION('',(-0.998629534754574,-0.0523359562429468,0.));
#14664=DIRECTION('center_axis',(0.,0.,-1.));
#14665=DIRECTION('ref_axis',(-0.309016994374952,0.951056516295152,0.));
#14666=DIRECTION('',(-0.951056516295152,-0.309016994374952,0.));
#14667=DIRECTION('',(-0.309016994374952,0.951056516295152,0.));
#14668=DIRECTION('',(0.951056516295152,0.309016994374952,0.));
#14669=DIRECTION('',(-0.777145961456968,-0.629320391049841,0.));
#14670=DIRECTION('center_axis',(0.,0.,-1.));
#14671=DIRECTION('ref_axis',(-0.809016994374951,0.587785252292469,0.));
#14672=DIRECTION('',(-0.587785252292468,-0.809016994374951,0.));
#14673=DIRECTION('',(-0.809016994374951,0.587785252292469,0.));
#14674=DIRECTION('',(0.587785252292469,0.809016994374951,0.));
#14675=DIRECTION('',(-0.258819045102522,-0.965925826289068,0.));
#14676=DIRECTION('center_axis',(0.,0.,-1.));
#14677=DIRECTION('ref_axis',(-1.,0.,0.));
#14678=DIRECTION('',(0.,-1.,0.));
#14679=DIRECTION('',(-1.,0.,0.));
#14680=DIRECTION('',(0.,1.,0.));
#14681=DIRECTION('',(0.358367949545307,-0.933580426497199,0.));
#14682=DIRECTION('center_axis',(0.,0.,-1.));
#14683=DIRECTION('ref_axis',(-0.809016994374942,-0.58778525229248,0.));
#14684=DIRECTION('',(0.58778525229248,-0.809016994374942,0.));
#14685=DIRECTION('',(-0.809016994374942,-0.58778525229248,0.));
#14686=DIRECTION('',(-0.58778525229248,0.809016994374942,0.));
#14687=DIRECTION('',(0.838670567945429,-0.54463903501502,0.));
#14688=DIRECTION('center_axis',(0.,0.,-1.));
#14689=DIRECTION('ref_axis',(-0.309016994374938,-0.951056516295157,0.));
#14690=DIRECTION('',(0.951056516295157,-0.309016994374938,0.));
#14691=DIRECTION('',(-0.309016994374938,-0.951056516295157,0.));
#14692=DIRECTION('',(-0.951056516295157,0.309016994374938,0.));
#14693=DIRECTION('',(0.998629534754573,0.0523359562429538,0.));
#14694=DIRECTION('center_axis',(0.,0.,-1.));
#14695=DIRECTION('ref_axis',(0.309016994374958,-0.95105651629515,0.));
#14696=DIRECTION('',(0.95105651629515,0.309016994374958,0.));
#14697=DIRECTION('',(0.309016994374958,-0.95105651629515,0.));
#14698=DIRECTION('',(-0.95105651629515,-0.309016994374958,0.));
#14699=DIRECTION('',(2.6394692217289E-16,1.,0.));
#14700=DIRECTION('',(2.6394692217289E-16,-1.,0.));
#14701=DIRECTION('',(-1.,0.,0.));
#14702=DIRECTION('center_axis',(0.,0.,1.));
#14703=DIRECTION('ref_axis',(1.,0.,0.));
#14704=DIRECTION('',(-2.6394692217289E-16,-1.,0.));
#14705=DIRECTION('',(1.,0.,0.));
#14706=DIRECTION('',(-2.6394692217289E-16,1.,0.));
#14707=DIRECTION('center_axis',(0.,0.,1.));
#14708=DIRECTION('ref_axis',(1.,0.,0.));
#14709=DIRECTION('center_axis',(0.,0.,1.));
#14710=DIRECTION('ref_axis',(1.,0.,0.));
#14711=DIRECTION('center_axis',(0.,1.,0.));
#14712=DIRECTION('ref_axis',(0.,0.,1.));
#14713=DIRECTION('',(0.,0.,-1.));
#14714=DIRECTION('',(-1.,0.,0.));
#14715=DIRECTION('',(0.,0.,-1.));
#14716=DIRECTION('center_axis',(-1.,0.,0.));
#14717=DIRECTION('ref_axis',(0.,0.,1.));
#14718=DIRECTION('center_axis',(1.,0.,0.));
#14719=DIRECTION('ref_axis',(0.,0.,1.));
#14720=DIRECTION('',(0.,0.,-1.));
#14721=DIRECTION('',(0.,1.,0.));
#14722=DIRECTION('center_axis',(0.,0.,-1.));
#14723=DIRECTION('ref_axis',(-1.,0.,0.));
#14724=DIRECTION('',(0.,0.,-1.));
#14725=DIRECTION('center_axis',(0.,0.,-1.));
#14726=DIRECTION('ref_axis',(1.,0.,0.));
#14727=DIRECTION('center_axis',(-0.965925826289068,0.258819045102522,0.));
#14728=DIRECTION('ref_axis',(-0.258819045102522,-0.965925826289068,0.));
#14729=DIRECTION('',(0.258819045102522,0.965925826289068,0.));
#14730=DIRECTION('center_axis',(1.,0.,0.));
#14731=DIRECTION('ref_axis',(0.,0.,-1.));
#14732=DIRECTION('center_axis',(-1.,0.,0.));
#14733=DIRECTION('ref_axis',(0.,0.,-1.));
#14734=DIRECTION('',(0.,-1.,0.));
#14735=DIRECTION('center_axis',(-1.,0.,0.));
#14736=DIRECTION('ref_axis',(0.,0.,1.));
#14737=DIRECTION('center_axis',(-0.587785252292474,0.809016994374947,0.));
#14738=DIRECTION('ref_axis',(-0.809016994374947,-0.587785252292474,0.));
#14739=DIRECTION('',(0.,0.,-1.));
#14740=DIRECTION('',(-0.809016994374947,-0.587785252292474,0.));
#14741=DIRECTION('',(0.,0.,-1.));
#14742=DIRECTION('center_axis',(-0.809016994374947,-0.587785252292474,0.));
#14743=DIRECTION('ref_axis',(0.587785252292474,-0.809016994374947,0.));
#14744=DIRECTION('center_axis',(0.809016994374947,0.587785252292474,0.));
#14745=DIRECTION('ref_axis',(0.587785252292474,-0.809016994374947,0.));
#14746=DIRECTION('',(0.,0.,-1.));
#14747=DIRECTION('',(-0.587785252292474,0.809016994374947,0.));
#14748=DIRECTION('center_axis',(0.,0.,-1.));
#14749=DIRECTION('ref_axis',(-1.,0.,0.));
#14750=DIRECTION('',(0.,0.,-1.));
#14751=DIRECTION('center_axis',(0.,0.,-1.));
#14752=DIRECTION('ref_axis',(0.809016994374947,0.587785252292474,0.));
#14753=DIRECTION('center_axis',(-0.933580426497202,-0.3583679495453,0.));
#14754=DIRECTION('ref_axis',(0.3583679495453,-0.933580426497202,0.));
#14755=DIRECTION('',(-0.3583679495453,0.933580426497202,0.));
#14756=DIRECTION('center_axis',(0.809016994374947,0.587785252292474,0.));
#14757=DIRECTION('ref_axis',(-0.587785252292474,0.809016994374947,0.));
#14758=DIRECTION('center_axis',(-0.809016994374947,-0.587785252292474,0.));
#14759=DIRECTION('ref_axis',(-0.587785252292474,0.809016994374947,0.));
#14760=DIRECTION('',(0.587785252292474,-0.809016994374947,0.));
#14761=DIRECTION('center_axis',(-0.951056516295155,0.309016994374945,0.));
#14762=DIRECTION('ref_axis',(-0.309016994374945,-0.951056516295155,0.));
#14763=DIRECTION('',(0.,0.,-1.));
#14764=DIRECTION('',(-0.309016994374945,-0.951056516295154,0.));
#14765=DIRECTION('',(0.,0.,-1.));
#14766=DIRECTION('center_axis',(-0.309016994374945,-0.951056516295155,0.));
#14767=DIRECTION('ref_axis',(0.951056516295155,-0.309016994374945,0.));
#14768=DIRECTION('center_axis',(0.309016994374945,0.951056516295155,0.));
#14769=DIRECTION('ref_axis',(0.951056516295154,-0.309016994374945,0.));
#14770=DIRECTION('',(0.,0.,-1.));
#14771=DIRECTION('',(-0.951056516295155,0.309016994374945,0.));
#14772=DIRECTION('center_axis',(0.,0.,-1.));
#14773=DIRECTION('ref_axis',(-1.,0.,0.));
#14774=DIRECTION('',(0.,0.,-1.));
#14775=DIRECTION('center_axis',(0.,0.,-1.));
#14776=DIRECTION('ref_axis',(0.309016994374945,0.951056516295154,0.));
#14777=DIRECTION('center_axis',(-0.544639035015026,-0.838670567945425,0.));
#14778=DIRECTION('ref_axis',(0.838670567945425,-0.544639035015026,0.));
#14779=DIRECTION('',(-0.838670567945425,0.544639035015026,0.));
#14780=DIRECTION('center_axis',(0.309016994374945,0.951056516295155,0.));
#14781=DIRECTION('ref_axis',(-0.951056516295155,0.309016994374945,0.));
#14782=DIRECTION('center_axis',(-0.309016994374945,-0.951056516295155,0.));
#14783=DIRECTION('ref_axis',(-0.951056516295154,0.309016994374945,0.));
#14784=DIRECTION('',(0.951056516295154,-0.309016994374945,0.));
#14785=DIRECTION('center_axis',(-0.951056516295152,-0.309016994374952,0.));
#14786=DIRECTION('ref_axis',(0.309016994374952,-0.951056516295152,0.));
#14787=DIRECTION('',(0.,0.,-1.));
#14788=DIRECTION('',(0.309016994374952,-0.951056516295152,0.));
#14789=DIRECTION('',(0.,0.,-1.));
#14790=DIRECTION('center_axis',(0.309016994374952,-0.951056516295152,0.));
#14791=DIRECTION('ref_axis',(0.951056516295152,0.309016994374952,0.));
#14792=DIRECTION('center_axis',(-0.309016994374952,0.951056516295152,0.));
#14793=DIRECTION('ref_axis',(0.951056516295152,0.309016994374952,0.));
#14794=DIRECTION('',(0.,0.,-1.));
#14795=DIRECTION('',(-0.951056516295152,-0.309016994374952,0.));
#14796=DIRECTION('center_axis',(0.,0.,-1.));
#14797=DIRECTION('ref_axis',(-1.,0.,0.));
#14798=DIRECTION('',(0.,0.,-1.));
#14799=DIRECTION('center_axis',(0.,0.,-1.));
#14800=DIRECTION('ref_axis',(-0.309016994374952,0.951056516295152,0.));
#14801=DIRECTION('center_axis',(0.0523359562429468,-0.998629534754574,0.));
#14802=DIRECTION('ref_axis',(0.998629534754574,0.0523359562429469,0.));
#14803=DIRECTION('',(-0.998629534754574,-0.0523359562429468,0.));
#14804=DIRECTION('center_axis',(-0.309016994374952,0.951056516295152,0.));
#14805=DIRECTION('ref_axis',(-0.951056516295152,-0.309016994374952,0.));
#14806=DIRECTION('center_axis',(0.309016994374952,-0.951056516295152,0.));
#14807=DIRECTION('ref_axis',(-0.951056516295152,-0.309016994374952,0.));
#14808=DIRECTION('',(0.951056516295152,0.309016994374952,0.));
#14809=DIRECTION('center_axis',(-0.587785252292469,-0.809016994374951,0.));
#14810=DIRECTION('ref_axis',(0.809016994374951,-0.587785252292469,0.));
#14811=DIRECTION('',(0.,0.,-1.));
#14812=DIRECTION('',(0.809016994374951,-0.587785252292468,0.));
#14813=DIRECTION('',(0.,0.,-1.));
#14814=DIRECTION('center_axis',(0.809016994374951,-0.587785252292469,0.));
#14815=DIRECTION('ref_axis',(0.587785252292469,0.809016994374951,0.));
#14816=DIRECTION('center_axis',(-0.809016994374951,0.587785252292469,0.));
#14817=DIRECTION('ref_axis',(0.587785252292469,0.809016994374951,0.));
#14818=DIRECTION('',(0.,0.,-1.));
#14819=DIRECTION('',(-0.587785252292469,-0.809016994374951,0.));
#14820=DIRECTION('center_axis',(0.,0.,-1.));
#14821=DIRECTION('ref_axis',(-1.,0.,0.));
#14822=DIRECTION('',(0.,0.,-1.));
#14823=DIRECTION('center_axis',(0.,0.,-1.));
#14824=DIRECTION('ref_axis',(-0.809016994374951,0.587785252292469,0.));
#14825=DIRECTION('center_axis',(0.629320391049841,-0.777145961456968,0.));
#14826=DIRECTION('ref_axis',(0.777145961456968,0.629320391049841,0.));
#14827=DIRECTION('',(-0.777145961456968,-0.629320391049841,0.));
#14828=DIRECTION('center_axis',(-0.809016994374951,0.587785252292469,0.));
#14829=DIRECTION('ref_axis',(-0.587785252292469,-0.809016994374951,0.));
#14830=DIRECTION('center_axis',(0.809016994374951,-0.587785252292469,0.));
#14831=DIRECTION('ref_axis',(-0.587785252292469,-0.809016994374951,0.));
#14832=DIRECTION('',(0.587785252292469,0.809016994374951,0.));
#14833=DIRECTION('center_axis',(0.,-1.,0.));
#14834=DIRECTION('ref_axis',(0.,0.,-1.));
#14835=DIRECTION('',(0.,0.,-1.));
#14836=DIRECTION('',(1.,0.,0.));
#14837=DIRECTION('',(0.,0.,-1.));
#14838=DIRECTION('center_axis',(1.,0.,0.));
#14839=DIRECTION('ref_axis',(0.,0.,-1.));
#14840=DIRECTION('center_axis',(-1.,0.,0.));
#14841=DIRECTION('ref_axis',(0.,0.,-1.));
#14842=DIRECTION('',(0.,0.,-1.));
#14843=DIRECTION('',(0.,-1.,0.));
#14844=DIRECTION('center_axis',(0.,0.,-1.));
#14845=DIRECTION('ref_axis',(-1.,0.,0.));
#14846=DIRECTION('',(0.,0.,-1.));
#14847=DIRECTION('center_axis',(0.,0.,-1.));
#14848=DIRECTION('ref_axis',(-1.,0.,0.));
#14849=DIRECTION('center_axis',(0.965925826289068,-0.258819045102522,0.));
#14850=DIRECTION('ref_axis',(0.258819045102522,0.965925826289068,0.));
#14851=DIRECTION('',(-0.258819045102522,-0.965925826289068,0.));
#14852=DIRECTION('center_axis',(-1.,0.,0.));
#14853=DIRECTION('ref_axis',(0.,0.,1.));
#14854=DIRECTION('center_axis',(1.,0.,0.));
#14855=DIRECTION('ref_axis',(0.,0.,1.));
#14856=DIRECTION('',(0.,1.,0.));
#14857=DIRECTION('center_axis',(0.58778525229248,-0.809016994374942,0.));
#14858=DIRECTION('ref_axis',(0.809016994374942,0.58778525229248,0.));
#14859=DIRECTION('',(0.,0.,-1.));
#14860=DIRECTION('',(0.809016994374942,0.58778525229248,0.));
#14861=DIRECTION('',(0.,0.,-1.));
#14862=DIRECTION('center_axis',(0.809016994374942,0.58778525229248,0.));
#14863=DIRECTION('ref_axis',(-0.58778525229248,0.809016994374942,0.));
#14864=DIRECTION('center_axis',(-0.809016994374942,-0.58778525229248,0.));
#14865=DIRECTION('ref_axis',(-0.58778525229248,0.809016994374942,0.));
#14866=DIRECTION('',(0.,0.,-1.));
#14867=DIRECTION('',(0.58778525229248,-0.809016994374942,0.));
#14868=DIRECTION('center_axis',(0.,0.,-1.));
#14869=DIRECTION('ref_axis',(-1.,0.,0.));
#14870=DIRECTION('',(0.,0.,-1.));
#14871=DIRECTION('center_axis',(0.,0.,-1.));
#14872=DIRECTION('ref_axis',(-0.809016994374942,-0.58778525229248,0.));
#14873=DIRECTION('center_axis',(0.933580426497199,0.358367949545307,0.));
#14874=DIRECTION('ref_axis',(-0.358367949545307,0.933580426497199,0.));
#14875=DIRECTION('',(0.358367949545307,-0.933580426497199,0.));
#14876=DIRECTION('center_axis',(-0.809016994374942,-0.58778525229248,0.));
#14877=DIRECTION('ref_axis',(0.58778525229248,-0.809016994374942,0.));
#14878=DIRECTION('center_axis',(0.809016994374942,0.58778525229248,0.));
#14879=DIRECTION('ref_axis',(0.58778525229248,-0.809016994374942,0.));
#14880=DIRECTION('',(-0.58778525229248,0.809016994374942,0.));
#14881=DIRECTION('center_axis',(0.951056516295157,-0.309016994374938,0.));
#14882=DIRECTION('ref_axis',(0.309016994374938,0.951056516295157,0.));
#14883=DIRECTION('',(0.,0.,-1.));
#14884=DIRECTION('',(0.309016994374938,0.951056516295157,0.));
#14885=DIRECTION('',(0.,0.,-1.));
#14886=DIRECTION('center_axis',(0.309016994374938,0.951056516295157,0.));
#14887=DIRECTION('ref_axis',(-0.951056516295157,0.309016994374938,0.));
#14888=DIRECTION('center_axis',(-0.309016994374938,-0.951056516295157,0.));
#14889=DIRECTION('ref_axis',(-0.951056516295157,0.309016994374938,0.));
#14890=DIRECTION('',(0.,0.,-1.));
#14891=DIRECTION('',(0.951056516295157,-0.309016994374938,0.));
#14892=DIRECTION('center_axis',(0.,0.,-1.));
#14893=DIRECTION('ref_axis',(-1.,0.,0.));
#14894=DIRECTION('',(0.,0.,-1.));
#14895=DIRECTION('center_axis',(0.,0.,-1.));
#14896=DIRECTION('ref_axis',(-0.309016994374938,-0.951056516295157,0.));
#14897=DIRECTION('center_axis',(0.54463903501502,0.838670567945429,0.));
#14898=DIRECTION('ref_axis',(-0.838670567945428,0.54463903501502,0.));
#14899=DIRECTION('',(0.838670567945429,-0.54463903501502,0.));
#14900=DIRECTION('center_axis',(-0.309016994374938,-0.951056516295157,0.));
#14901=DIRECTION('ref_axis',(0.951056516295157,-0.309016994374938,0.));
#14902=DIRECTION('center_axis',(0.309016994374938,0.951056516295157,0.));
#14903=DIRECTION('ref_axis',(0.951056516295157,-0.309016994374938,0.));
#14904=DIRECTION('',(-0.951056516295157,0.309016994374938,0.));
#14905=DIRECTION('center_axis',(0.95105651629515,0.309016994374958,0.));
#14906=DIRECTION('ref_axis',(-0.309016994374958,0.95105651629515,0.));
#14907=DIRECTION('',(0.,0.,-1.));
#14908=DIRECTION('',(-0.309016994374958,0.95105651629515,0.));
#14909=DIRECTION('',(0.,0.,-1.));
#14910=DIRECTION('center_axis',(-0.309016994374958,0.95105651629515,0.));
#14911=DIRECTION('ref_axis',(-0.95105651629515,-0.309016994374958,0.));
#14912=DIRECTION('center_axis',(0.309016994374958,-0.95105651629515,0.));
#14913=DIRECTION('ref_axis',(-0.95105651629515,-0.309016994374958,0.));
#14914=DIRECTION('',(0.,0.,-1.));
#14915=DIRECTION('',(0.95105651629515,0.309016994374958,0.));
#14916=DIRECTION('center_axis',(0.,0.,-1.));
#14917=DIRECTION('ref_axis',(-1.,0.,0.));
#14918=DIRECTION('',(0.,0.,-1.));
#14919=DIRECTION('center_axis',(0.,0.,-1.));
#14920=DIRECTION('ref_axis',(0.309016994374958,-0.95105651629515,0.));
#14921=DIRECTION('center_axis',(-0.0523359562429538,0.998629534754573,0.));
#14922=DIRECTION('ref_axis',(-0.998629534754574,-0.0523359562429538,0.));
#14923=DIRECTION('',(0.998629534754573,0.0523359562429538,0.));
#14924=DIRECTION('center_axis',(0.309016994374958,-0.95105651629515,0.));
#14925=DIRECTION('ref_axis',(0.95105651629515,0.309016994374958,0.));
#14926=DIRECTION('center_axis',(-0.309016994374958,0.95105651629515,0.));
#14927=DIRECTION('ref_axis',(0.95105651629515,0.309016994374958,0.));
#14928=DIRECTION('',(-0.95105651629515,-0.309016994374958,0.));
#14929=DIRECTION('center_axis',(0.587785252292463,0.809016994374955,0.));
#14930=DIRECTION('ref_axis',(-0.809016994374955,0.587785252292463,0.));
#14931=DIRECTION('',(0.,0.,-1.));
#14932=DIRECTION('',(-0.809016994374955,0.587785252292463,0.));
#14933=DIRECTION('',(0.,0.,-1.));
#14934=DIRECTION('center_axis',(-0.809016994374955,0.587785252292462,0.));
#14935=DIRECTION('ref_axis',(-0.587785252292462,-0.809016994374955,0.));
#14936=DIRECTION('center_axis',(0.809016994374955,-0.587785252292462,0.));
#14937=DIRECTION('ref_axis',(-0.587785252292462,-0.809016994374955,0.));
#14938=DIRECTION('',(0.,0.,-1.));
#14939=DIRECTION('',(0.587785252292462,0.809016994374955,0.));
#14940=DIRECTION('center_axis',(0.,0.,-1.));
#14941=DIRECTION('ref_axis',(-1.,0.,0.));
#14942=DIRECTION('',(0.,0.,-1.));
#14943=DIRECTION('center_axis',(0.,0.,-1.));
#14944=DIRECTION('ref_axis',(0.809016994374955,-0.587785252292462,0.));
#14945=DIRECTION('center_axis',(-0.629320391049847,0.777145961456963,0.));
#14946=DIRECTION('ref_axis',(-0.777145961456964,-0.629320391049847,0.));
#14947=DIRECTION('',(0.777145961456963,0.629320391049847,0.));
#14948=DIRECTION('center_axis',(0.809016994374955,-0.587785252292463,0.));
#14949=DIRECTION('ref_axis',(0.587785252292463,0.809016994374955,0.));
#14950=DIRECTION('center_axis',(-0.809016994374955,0.587785252292463,0.));
#14951=DIRECTION('ref_axis',(0.587785252292463,0.809016994374955,0.));
#14952=DIRECTION('',(-0.587785252292463,-0.809016994374955,0.));
#14953=DIRECTION('center_axis',(-0.809016994374947,-0.587785252292474,0.));
#14954=DIRECTION('ref_axis',(0.587785252292474,-0.809016994374947,0.));
#14955=DIRECTION('center_axis',(-0.309016994374945,-0.951056516295155,0.));
#14956=DIRECTION('ref_axis',(0.951056516295155,-0.309016994374945,0.));
#14957=DIRECTION('center_axis',(0.309016994374952,-0.951056516295152,0.));
#14958=DIRECTION('ref_axis',(0.951056516295152,0.309016994374952,0.));
#14959=DIRECTION('center_axis',(0.809016994374951,-0.587785252292469,0.));
#14960=DIRECTION('ref_axis',(0.587785252292469,0.809016994374951,0.));
#14961=DIRECTION('center_axis',(1.,0.,0.));
#14962=DIRECTION('ref_axis',(0.,0.,-1.));
#14963=DIRECTION('center_axis',(0.809016994374942,0.58778525229248,0.));
#14964=DIRECTION('ref_axis',(-0.58778525229248,0.809016994374942,0.));
#14965=DIRECTION('center_axis',(0.309016994374938,0.951056516295157,0.));
#14966=DIRECTION('ref_axis',(-0.951056516295157,0.309016994374938,0.));
#14967=DIRECTION('center_axis',(-0.309016994374958,0.95105651629515,0.));
#14968=DIRECTION('ref_axis',(-0.95105651629515,-0.309016994374958,0.));
#14969=DIRECTION('center_axis',(-0.809016994374955,0.587785252292463,0.));
#14970=DIRECTION('ref_axis',(-0.587785252292462,-0.809016994374955,0.));
#14971=DIRECTION('center_axis',(0.,0.,1.));
#14972=DIRECTION('ref_axis',(1.,0.,0.));
#14973=DIRECTION('center_axis',(0.,0.,1.));
#14974=DIRECTION('ref_axis',(1.,0.,0.));
#14975=DIRECTION('center_axis',(0.,0.,1.));
#14976=DIRECTION('ref_axis',(1.,0.,0.));
#14977=DIRECTION('center_axis',(0.,0.,1.));
#14978=DIRECTION('ref_axis',(1.,0.,0.));
#14979=DIRECTION('center_axis',(0.,0.,1.));
#14980=DIRECTION('ref_axis',(1.,0.,0.));
#14981=DIRECTION('center_axis',(0.,0.,1.));
#14982=DIRECTION('ref_axis',(1.,0.,0.));
#14983=DIRECTION('center_axis',(0.,0.,1.));
#14984=DIRECTION('ref_axis',(1.,0.,0.));
#14985=DIRECTION('center_axis',(0.,0.,1.));
#14986=DIRECTION('ref_axis',(1.,0.,0.));
#14987=DIRECTION('center_axis',(0.,0.,1.));
#14988=DIRECTION('ref_axis',(1.,0.,0.));
#14989=DIRECTION('center_axis',(0.,0.,1.));
#14990=DIRECTION('ref_axis',(1.,0.,0.));
#14991=DIRECTION('center_axis',(0.,0.,1.));
#14992=DIRECTION('ref_axis',(1.,0.,0.));
#14993=DIRECTION('center_axis',(1.,-2.6394692217289E-16,0.));
#14994=DIRECTION('ref_axis',(2.6394692217289E-16,1.,0.));
#14995=DIRECTION('',(0.,0.,-1.));
#14996=DIRECTION('center_axis',(0.,1.,0.));
#14997=DIRECTION('ref_axis',(0.,0.,1.));
#14998=DIRECTION('',(0.,0.,-1.));
#14999=DIRECTION('center_axis',(-1.,-2.6394692217289E-16,0.));
#15000=DIRECTION('ref_axis',(2.6394692217289E-16,-1.,0.));
#25203=CARTESIAN_POINT('',(0.,0.,0.));
#25204=CARTESIAN_POINT('Origin',(0.,0.,137.5));
#25205=CARTESIAN_POINT('',(-37.0000000000001,-4.53119315684522E-15,137.5));
#25206=CARTESIAN_POINT('Origin',(0.,0.,137.5));
#25207=CARTESIAN_POINT('',(-35.,-4.28626379701574E-15,135.5));
#25208=CARTESIAN_POINT('',(-37.0000000000001,-4.53119315684522E-15,137.5));
#25209=CARTESIAN_POINT('',(35.,4.28626379701574E-15,135.5));
#25210=CARTESIAN_POINT('Origin',(0.,0.,135.5));
#25211=CARTESIAN_POINT('Origin',(0.,0.,135.5));
#25212=CARTESIAN_POINT('Origin',(0.,0.,0.999999999999973));
#25213=CARTESIAN_POINT('',(30.,3.67394039744206E-15,0.999999999999973));
#25214=CARTESIAN_POINT('',(-30.,-3.67394039744206E-15,0.999999999999973));
#25215=CARTESIAN_POINT('Origin',(0.,0.,0.999999999999973));
#25216=CARTESIAN_POINT('Origin',(0.,0.,0.999999999999973));
#25217=CARTESIAN_POINT('',(-29.0000000000001,-3.55147571752733E-15,1.38777878078145E-16));
#25218=CARTESIAN_POINT('',(-30.,-3.67394039744206E-15,0.999999999999973));
#25219=CARTESIAN_POINT('Origin',(0.,0.,0.));
#25220=CARTESIAN_POINT('Origin',(0.,0.,88.4999999999999));
#25221=CARTESIAN_POINT('',(35.,4.28626379701574E-15,88.4999999999999));
#25222=CARTESIAN_POINT('',(-35.,-4.28626379701574E-15,88.4999999999999));
#25223=CARTESIAN_POINT('Origin',(0.,0.,88.4999999999999));
#25224=CARTESIAN_POINT('Origin',(0.,0.,88.4999999999999));
#25225=CARTESIAN_POINT('',(-34.0000000000001,-4.16379911710102E-15,87.5));
#25226=CARTESIAN_POINT('',(-35.,-4.28626379701574E-15,88.4999999999999));
#25227=CARTESIAN_POINT('Origin',(0.,0.,87.5));
#25228=CARTESIAN_POINT('Origin',(0.,0.,342.5));
#25229=CARTESIAN_POINT('',(-3.,9.01387818865997,150.));
#25230=CARTESIAN_POINT('',(3.,9.01387818865997,150.));
#25231=CARTESIAN_POINT('Origin',(0.,0.,150.));
#25232=CARTESIAN_POINT('',(3.,9.01387818865997,0.));
#25233=CARTESIAN_POINT('',(3.,9.01387818865997,342.5));
#25234=CARTESIAN_POINT('',(-3.,9.01387818865997,0.));
#25235=CARTESIAN_POINT('Origin',(0.,0.,0.));
#25236=CARTESIAN_POINT('',(-3.,9.01387818865997,342.5));
#25237=CARTESIAN_POINT('Origin',(0.,0.,342.5));
#25238=CARTESIAN_POINT('',(120.,-1.46957615897682E-14,342.5));
#25239=CARTESIAN_POINT('Origin',(0.,0.,342.5));
#25240=CARTESIAN_POINT('',(120.,-1.46957615897682E-14,330.));
#25241=CARTESIAN_POINT('',(120.,-1.46957615897682E-14,342.5));
#25242=CARTESIAN_POINT('',(114.126781955419,-37.0820393249926,330.));
#25243=CARTESIAN_POINT('Origin',(0.,0.,330.));
#25244=CARTESIAN_POINT('',(112.827292588217,-40.8656585314966,330.));
#25245=CARTESIAN_POINT('Origin',(0.,0.,330.));
#25246=CARTESIAN_POINT('',(70.5342302750976,-97.0820393249931,330.));
#25247=CARTESIAN_POINT('Origin',(0.,0.,330.));
#25248=CARTESIAN_POINT('',(67.2589657231482,-99.3792308777461,330.));
#25249=CARTESIAN_POINT('Origin',(0.,0.,330.));
#25250=CARTESIAN_POINT('',(0.,-120.,330.));
#25251=CARTESIAN_POINT('Origin',(0.,0.,330.));
#25252=CARTESIAN_POINT('',(-4.,-119.93331480452,330.));
#25253=CARTESIAN_POINT('Origin',(0.,0.,330.));
#25254=CARTESIAN_POINT('',(-70.5342302750962,-97.0820393249941,330.));
#25255=CARTESIAN_POINT('Origin',(0.,0.,330.));
#25256=CARTESIAN_POINT('',(-73.7311016781464,-94.6769488594074,330.));
#25257=CARTESIAN_POINT('Origin',(0.,0.,330.));
#25258=CARTESIAN_POINT('',(-114.126781955418,-37.0820393249942,330.));
#25259=CARTESIAN_POINT('Origin',(0.,0.,330.));
#25260=CARTESIAN_POINT('',(-115.299428543216,-33.2572064011369,330.));
#25261=CARTESIAN_POINT('Origin',(0.,0.,330.));
#25262=CARTESIAN_POINT('',(-114.126781955419,37.0820393249934,330.));
#25263=CARTESIAN_POINT('Origin',(0.,0.,330.));
#25264=CARTESIAN_POINT('',(-112.827292588217,40.8656585314973,330.));
#25265=CARTESIAN_POINT('Origin',(0.,0.,330.));
#25266=CARTESIAN_POINT('',(-70.5342302750969,97.0820393249936,330.));
#25267=CARTESIAN_POINT('Origin',(0.,0.,330.));
#25268=CARTESIAN_POINT('',(-67.2589657231475,99.3792308777467,330.));
#25269=CARTESIAN_POINT('Origin',(0.,0.,330.));
#25270=CARTESIAN_POINT('',(0.,120.,330.));
#25271=CARTESIAN_POINT('Origin',(0.,0.,330.));
#25272=CARTESIAN_POINT('',(4.,119.93331480452,330.));
#25273=CARTESIAN_POINT('Origin',(0.,0.,330.));
#25274=CARTESIAN_POINT('',(70.5342302750955,97.0820393249946,330.));
#25275=CARTESIAN_POINT('Origin',(0.,0.,330.));
#25276=CARTESIAN_POINT('',(73.7311016781457,94.6769488594079,330.));
#25277=CARTESIAN_POINT('Origin',(0.,0.,330.));
#25278=CARTESIAN_POINT('',(114.126781955418,37.082039324995,330.));
#25279=CARTESIAN_POINT('Origin',(0.,0.,330.));
#25280=CARTESIAN_POINT('',(115.299428543216,33.2572064011377,330.));
#25281=CARTESIAN_POINT('Origin',(0.,0.,330.));
#25282=CARTESIAN_POINT('Origin',(0.,0.,330.));
#25283=CARTESIAN_POINT('Origin',(0.,0.,150.));
#25284=CARTESIAN_POINT('',(160.,-1.95943487863577E-14,137.5));
#25285=CARTESIAN_POINT('Origin',(0.,0.,137.5));
#25286=CARTESIAN_POINT('',(160.,-1.95943487863577E-14,150.));
#25287=CARTESIAN_POINT('',(160.,-1.95943487863577E-14,150.));
#25288=CARTESIAN_POINT('',(152.169042607225,-49.4427190999901,150.));
#25289=CARTESIAN_POINT('Origin',(0.,0.,150.));
#25290=CARTESIAN_POINT('',(152.169042607225,-49.4427190999901,330.));
#25291=CARTESIAN_POINT('',(152.169042607225,-49.4427190999901,330.));
#25292=CARTESIAN_POINT('',(160.,-1.95943487863577E-14,330.));
#25293=CARTESIAN_POINT('Origin',(0.,0.,330.));
#25294=CARTESIAN_POINT('',(160.,-1.95943487863577E-14,342.5));
#25295=CARTESIAN_POINT('',(160.,-1.95943487863577E-14,150.));
#25296=CARTESIAN_POINT('Origin',(0.,0.,342.5));
#25297=CARTESIAN_POINT('',(159.780725560732,8.37375299887273,330.));
#25298=CARTESIAN_POINT('Origin',(0.,0.,330.));
#25299=CARTESIAN_POINT('',(159.780725560732,8.37375299887273,150.));
#25300=CARTESIAN_POINT('',(159.780725560732,8.37375299887273,330.));
#25301=CARTESIAN_POINT('Origin',(0.,0.,150.));
#25302=CARTESIAN_POINT('',(-152.169042607225,49.4427190999912,330.));
#25303=CARTESIAN_POINT('',(-159.780725560732,-8.37375299887161,330.));
#25304=CARTESIAN_POINT('Origin',(0.,0.,330.));
#25305=CARTESIAN_POINT('',(-159.780725560732,-8.37375299887161,150.));
#25306=CARTESIAN_POINT('',(-159.780725560732,-8.37375299887161,330.));
#25307=CARTESIAN_POINT('',(-152.169042607225,49.4427190999912,150.));
#25308=CARTESIAN_POINT('Origin',(0.,0.,150.));
#25309=CARTESIAN_POINT('',(-152.169042607225,49.4427190999912,330.));
#25310=CARTESIAN_POINT('',(94.0456403667969,-129.442719099991,330.));
#25311=CARTESIAN_POINT('',(94.0456403667969,-129.442719099991,150.));
#25312=CARTESIAN_POINT('',(94.0456403667969,-129.442719099991,330.));
#25313=CARTESIAN_POINT('',(134.187290871269,-87.1422456024031,330.));
#25314=CARTESIAN_POINT('Origin',(0.,0.,330.));
#25315=CARTESIAN_POINT('',(134.187290871269,-87.1422456024031,150.));
#25316=CARTESIAN_POINT('',(134.187290871269,-87.1422456024031,330.));
#25317=CARTESIAN_POINT('Origin',(0.,0.,150.));
#25318=CARTESIAN_POINT('',(0.,-160.,330.));
#25319=CARTESIAN_POINT('',(0.,-160.,150.));
#25320=CARTESIAN_POINT('',(0.,-160.,330.));
#25321=CARTESIAN_POINT('',(57.3388719272493,-149.372868239552,330.));
#25322=CARTESIAN_POINT('Origin',(0.,0.,330.));
#25323=CARTESIAN_POINT('',(57.3388719272493,-149.372868239552,150.));
#25324=CARTESIAN_POINT('',(57.3388719272493,-149.372868239552,330.));
#25325=CARTESIAN_POINT('Origin',(0.,0.,150.));
#25326=CARTESIAN_POINT('',(-94.045640366795,-129.442719099992,330.));
#25327=CARTESIAN_POINT('',(-94.045640366795,-129.442719099992,150.));
#25328=CARTESIAN_POINT('',(-94.045640366795,-129.442719099992,330.));
#25329=CARTESIAN_POINT('',(-41.4110472164034,-154.548132206251,330.));
#25330=CARTESIAN_POINT('Origin',(0.,0.,330.));
#25331=CARTESIAN_POINT('',(-41.4110472164034,-154.548132206251,150.));
#25332=CARTESIAN_POINT('',(-41.4110472164034,-154.548132206251,330.));
#25333=CARTESIAN_POINT('Origin',(0.,0.,150.));
#25334=CARTESIAN_POINT('',(-152.169042607224,-49.4427190999923,330.));
#25335=CARTESIAN_POINT('',(-152.169042607224,-49.4427190999923,150.));
#25336=CARTESIAN_POINT('',(-152.169042607224,-49.4427190999923,330.));
#25337=CARTESIAN_POINT('',(-124.343353833115,-100.691262567975,330.));
#25338=CARTESIAN_POINT('Origin',(0.,0.,330.));
#25339=CARTESIAN_POINT('',(-124.343353833115,-100.691262567975,150.));
#25340=CARTESIAN_POINT('',(-124.343353833115,-100.691262567975,330.));
#25341=CARTESIAN_POINT('Origin',(0.,0.,150.));
#25342=CARTESIAN_POINT('',(94.045640366794,129.442719099993,330.));
#25343=CARTESIAN_POINT('',(41.4110472164034,154.548132206251,330.));
#25344=CARTESIAN_POINT('Origin',(0.,0.,330.));
#25345=CARTESIAN_POINT('',(41.4110472164034,154.548132206251,150.));
#25346=CARTESIAN_POINT('',(41.4110472164034,154.548132206251,330.));
#25347=CARTESIAN_POINT('',(94.045640366794,129.442719099993,150.));
#25348=CARTESIAN_POINT('Origin',(0.,0.,150.));
#25349=CARTESIAN_POINT('',(94.045640366794,129.442719099993,330.));
#25350=CARTESIAN_POINT('',(152.169042607224,49.4427190999933,330.));
#25351=CARTESIAN_POINT('',(152.169042607224,49.4427190999933,150.));
#25352=CARTESIAN_POINT('',(152.169042607224,49.4427190999933,330.));
#25353=CARTESIAN_POINT('',(124.343353833114,100.691262567976,330.));
#25354=CARTESIAN_POINT('Origin',(0.,0.,330.));
#25355=CARTESIAN_POINT('',(124.343353833114,100.691262567976,150.));
#25356=CARTESIAN_POINT('',(124.343353833114,100.691262567976,330.));
#25357=CARTESIAN_POINT('Origin',(0.,0.,150.));
#25358=CARTESIAN_POINT('',(-94.0456403667959,129.442719099992,330.));
#25359=CARTESIAN_POINT('',(-94.0456403667959,129.442719099991,150.));
#25360=CARTESIAN_POINT('',(-94.0456403667959,129.442719099992,330.));
#25361=CARTESIAN_POINT('',(-134.187290871268,87.142245602404,330.));
#25362=CARTESIAN_POINT('Origin',(0.,0.,330.));
#25363=CARTESIAN_POINT('',(-134.187290871268,87.142245602404,150.));
#25364=CARTESIAN_POINT('',(-134.187290871268,87.142245602404,330.));
#25365=CARTESIAN_POINT('Origin',(0.,0.,150.));
#25366=CARTESIAN_POINT('',(0.,160.,330.));
#25367=CARTESIAN_POINT('',(0.,160.,150.));
#25368=CARTESIAN_POINT('',(0.,160.,330.));
#25369=CARTESIAN_POINT('',(-57.3388719272482,149.372868239552,330.));
#25370=CARTESIAN_POINT('Origin',(0.,0.,330.));
#25371=CARTESIAN_POINT('',(-57.3388719272482,149.372868239552,150.));
#25372=CARTESIAN_POINT('',(-57.3388719272482,149.372868239552,330.));
#25373=CARTESIAN_POINT('Origin',(0.,0.,150.));
#25374=CARTESIAN_POINT('Origin',(0.,0.,137.5));
#25375=CARTESIAN_POINT('',(35.,-4.28626379701574E-15,137.5));
#25376=CARTESIAN_POINT('Origin',(0.,0.,87.5));
#25377=CARTESIAN_POINT('',(30.,-3.67394039744206E-15,87.5));
#25378=CARTESIAN_POINT('',(30.,-3.67394039744206E-15,87.5));
#25379=CARTESIAN_POINT('Origin',(0.,0.,87.5));
#25380=CARTESIAN_POINT('Origin',(0.,0.,330.));
#25381=CARTESIAN_POINT('',(0.,105.,330.));
#25382=CARTESIAN_POINT('',(0.,95.,330.));
#25383=CARTESIAN_POINT('',(4.,105.,330.));
#25384=CARTESIAN_POINT('',(4.,105.,330.));
#25385=CARTESIAN_POINT('',(4.,95.,330.));
#25386=CARTESIAN_POINT('Origin',(0.,0.,330.));
#25387=CARTESIAN_POINT('',(-61.7174514907098,84.9467844093694,330.));
#25388=CARTESIAN_POINT('',(-55.8395989677851,76.85661446562,330.));
#25389=CARTESIAN_POINT('',(-58.48138351321,87.2979254185393,330.));
#25390=CARTESIAN_POINT('',(-58.48138351321,87.2979254185393,330.));
#25391=CARTESIAN_POINT('',(-52.6035309902853,79.2077554747898,330.));
#25392=CARTESIAN_POINT('Origin',(0.,0.,330.));
#25393=CARTESIAN_POINT('',(-99.8609342109912,32.4467844093692,330.));
#25394=CARTESIAN_POINT('',(-90.3503690480397,29.3566144656198,330.));
#25395=CARTESIAN_POINT('',(-98.6248662334914,36.2510104745498,330.));
#25396=CARTESIAN_POINT('',(-98.6248662334914,36.2510104745498,330.));
#25397=CARTESIAN_POINT('',(-89.1143010705399,33.1608405308004,330.));
#25398=CARTESIAN_POINT('Origin',(0.,0.,330.));
#25399=CARTESIAN_POINT('',(-99.860934210991,-32.4467844093699,330.));
#25400=CARTESIAN_POINT('',(-90.3503690480395,-29.3566144656204,330.));
#25401=CARTESIAN_POINT('',(-101.097002188491,-28.6425583441893,330.));
#25402=CARTESIAN_POINT('',(-101.097002188491,-28.6425583441893,330.));
#25403=CARTESIAN_POINT('',(-91.5864370255393,-25.5523884004398,330.));
#25404=CARTESIAN_POINT('Origin',(0.,0.,330.));
#25405=CARTESIAN_POINT('',(-61.7174514907092,-84.9467844093698,330.));
#25406=CARTESIAN_POINT('',(-55.8395989677845,-76.8566144656203,330.));
#25407=CARTESIAN_POINT('',(-64.953519468209,-82.5956434001999,330.));
#25408=CARTESIAN_POINT('',(-64.953519468209,-82.5956434001999,330.));
#25409=CARTESIAN_POINT('',(-59.0756669452843,-74.5054734564505,330.));
#25410=CARTESIAN_POINT('Origin',(0.,0.,330.));
#25411=CARTESIAN_POINT('',(0.,-105.,330.));
#25412=CARTESIAN_POINT('',(0.,-95.,330.));
#25413=CARTESIAN_POINT('',(-4.,-105.,330.));
#25414=CARTESIAN_POINT('',(-4.,-105.,330.));
#25415=CARTESIAN_POINT('',(-4.,-95.,330.));
#25416=CARTESIAN_POINT('Origin',(0.,0.,330.));
#25417=CARTESIAN_POINT('',(61.7174514907104,-84.9467844093689,330.));
#25418=CARTESIAN_POINT('',(55.8395989677856,-76.8566144656195,330.));
#25419=CARTESIAN_POINT('',(58.4813835132107,-87.2979254185389,330.));
#25420=CARTESIAN_POINT('',(58.4813835132107,-87.2979254185389,330.));
#25421=CARTESIAN_POINT('',(52.6035309902859,-79.2077554747894,330.));
#25422=CARTESIAN_POINT('Origin',(0.,0.,330.));
#25423=CARTESIAN_POINT('',(99.8609342109914,-32.4467844093685,330.));
#25424=CARTESIAN_POINT('',(90.3503690480399,-29.3566144656191,330.));
#25425=CARTESIAN_POINT('',(98.6248662334917,-36.2510104745491,330.));
#25426=CARTESIAN_POINT('',(98.6248662334917,-36.2510104745491,330.));
#25427=CARTESIAN_POINT('',(89.1143010705401,-33.1608405307998,330.));
#25428=CARTESIAN_POINT('Origin',(0.,0.,330.));
#25429=CARTESIAN_POINT('',(99.8609342109908,32.4467844093706,330.));
#25430=CARTESIAN_POINT('',(90.3503690480393,29.356614465621,330.));
#25431=CARTESIAN_POINT('',(101.097002188491,28.64255834419,330.));
#25432=CARTESIAN_POINT('',(101.097002188491,28.64255834419,330.));
#25433=CARTESIAN_POINT('',(91.5864370255391,25.5523884004404,330.));
#25434=CARTESIAN_POINT('Origin',(0.,0.,330.));
#25435=CARTESIAN_POINT('',(61.7174514907085,84.9467844093703,330.));
#25436=CARTESIAN_POINT('',(55.8395989677839,76.8566144656207,330.));
#25437=CARTESIAN_POINT('',(64.9535194682084,82.5956434002004,330.));
#25438=CARTESIAN_POINT('',(64.9535194682084,82.5956434002004,330.));
#25439=CARTESIAN_POINT('',(59.0756669452838,74.5054734564509,330.));
#25440=CARTESIAN_POINT('Origin',(0.,0.,150.));
#25441=CARTESIAN_POINT('',(121.234769987286,98.1739810037762,150.));
#25442=CARTESIAN_POINT('',(124.343353833114,100.691262567976,150.));
#25443=CARTESIAN_POINT('',(94.9004195456003,123.814015240881,150.));
#25444=CARTESIAN_POINT('Origin',(0.,0.,150.));
#25445=CARTESIAN_POINT('',(59.0756669452838,74.5054734564509,150.));
#25446=CARTESIAN_POINT('',(59.0756669452838,74.5054734564509,150.));
#25447=CARTESIAN_POINT('',(55.8395989677839,76.8566144656207,150.));
#25448=CARTESIAN_POINT('',(55.8395989677839,76.8566144656207,150.));
#25449=CARTESIAN_POINT('',(55.8395989677839,76.8566144656207,150.));
#25450=CARTESIAN_POINT('',(40.3757710359933,150.684428901095,150.));
#25451=CARTESIAN_POINT('',(41.4110472164034,154.548132206251,150.));
#25452=CARTESIAN_POINT('',(4.00000000000002,155.948709516943,150.));
#25453=CARTESIAN_POINT('Origin',(0.,0.,150.));
#25454=CARTESIAN_POINT('',(4.,95.,150.));
#25455=CARTESIAN_POINT('',(4.,95.,150.));
#25456=CARTESIAN_POINT('',(0.,95.,150.));
#25457=CARTESIAN_POINT('',(0.,95.,150.));
#25458=CARTESIAN_POINT('',(0.,95.,150.));
#25459=CARTESIAN_POINT('',(-55.905400129067,145.638546533563,150.));
#25460=CARTESIAN_POINT('',(-57.3388719272482,149.372868239552,150.));
#25461=CARTESIAN_POINT('',(-88.4282835906026,128.516297259219,150.));
#25462=CARTESIAN_POINT('Origin',(0.,0.,150.));
#25463=CARTESIAN_POINT('',(-52.6035309902853,79.2077554747898,150.));
#25464=CARTESIAN_POINT('',(-52.6035309902853,79.2077554747898,150.));
#25465=CARTESIAN_POINT('',(-55.8395989677851,76.85661446562,150.));
#25466=CARTESIAN_POINT('',(-55.8395989677851,76.85661446562,150.));
#25467=CARTESIAN_POINT('',(-55.8395989677851,76.85661446562,150.));
#25468=CARTESIAN_POINT('',(-130.832608599486,84.963689462344,150.));
#25469=CARTESIAN_POINT('',(-134.187290871268,87.142245602404,150.));
#25470=CARTESIAN_POINT('',(-147.079968416409,51.9950275567578,150.));
#25471=CARTESIAN_POINT('Origin',(0.,0.,150.));
#25472=CARTESIAN_POINT('',(-89.1143010705399,33.1608405308004,150.));
#25473=CARTESIAN_POINT('',(-89.1143010705399,33.1608405308004,150.));
#25474=CARTESIAN_POINT('',(-90.3503690480397,29.3566144656197,150.));
#25475=CARTESIAN_POINT('',(-90.3503690480397,29.3566144656198,150.));
#25476=CARTESIAN_POINT('',(-90.3503690480397,29.3566144656198,150.));
#25477=CARTESIAN_POINT('',(-155.786207421714,-8.16440917389982,150.));
#25478=CARTESIAN_POINT('',(-159.780725560732,-8.37375299887161,150.));
#25479=CARTESIAN_POINT('',(-149.552104371409,-44.3865754263977,150.));
#25480=CARTESIAN_POINT('Origin',(0.,0.,150.));
#25481=CARTESIAN_POINT('',(-91.5864370255393,-25.5523884004398,150.));
#25482=CARTESIAN_POINT('',(-91.5864370255393,-25.5523884004398,150.));
#25483=CARTESIAN_POINT('',(-90.3503690480395,-29.3566144656204,150.));
#25484=CARTESIAN_POINT('',(-90.3503690480395,-29.3566144656204,150.));
#25485=CARTESIAN_POINT('',(-90.3503690480395,-29.3566144656204,150.));
#25486=CARTESIAN_POINT('',(-121.234769987287,-98.1739810037753,150.));
#25487=CARTESIAN_POINT('',(-124.343353833115,-100.691262567975,150.));
#25488=CARTESIAN_POINT('',(-94.9004195456013,-123.81401524088,150.));
#25489=CARTESIAN_POINT('Origin',(0.,0.,150.));
#25490=CARTESIAN_POINT('',(-59.0756669452843,-74.5054734564505,150.));
#25491=CARTESIAN_POINT('',(-59.0756669452843,-74.5054734564505,150.));
#25492=CARTESIAN_POINT('',(-55.8395989677845,-76.8566144656203,150.));
#25493=CARTESIAN_POINT('',(-55.8395989677845,-76.8566144656203,150.));
#25494=CARTESIAN_POINT('',(-55.8395989677845,-76.8566144656203,150.));
#25495=CARTESIAN_POINT('',(-40.3757710359933,-150.684428901095,150.));
#25496=CARTESIAN_POINT('',(-41.4110472164034,-154.548132206251,150.));
#25497=CARTESIAN_POINT('',(-4.,-155.948709516943,150.));
#25498=CARTESIAN_POINT('Origin',(0.,0.,150.));
#25499=CARTESIAN_POINT('',(-4.,-95.,150.));
#25500=CARTESIAN_POINT('',(-4.,-95.,150.));
#25501=CARTESIAN_POINT('',(0.,-95.,150.));
#25502=CARTESIAN_POINT('',(0.,-95.,150.));
#25503=CARTESIAN_POINT('',(0.,-95.,150.));
#25504=CARTESIAN_POINT('',(55.905400129068,-145.638546533563,150.));
#25505=CARTESIAN_POINT('',(57.3388719272493,-149.372868239552,150.));
#25506=CARTESIAN_POINT('',(88.4282835906036,-128.516297259218,150.));
#25507=CARTESIAN_POINT('Origin',(0.,0.,150.));
#25508=CARTESIAN_POINT('',(52.6035309902859,-79.2077554747895,150.));
#25509=CARTESIAN_POINT('',(52.6035309902859,-79.2077554747894,150.));
#25510=CARTESIAN_POINT('',(55.8395989677856,-76.8566144656195,150.));
#25511=CARTESIAN_POINT('',(55.8395989677856,-76.8566144656195,150.));
#25512=CARTESIAN_POINT('',(55.8395989677856,-76.8566144656195,150.));
#25513=CARTESIAN_POINT('',(130.832608599487,-84.9636894623431,150.));
#25514=CARTESIAN_POINT('',(134.187290871269,-87.1422456024031,150.));
#25515=CARTESIAN_POINT('',(147.07996841641,-51.9950275567568,150.));
#25516=CARTESIAN_POINT('Origin',(0.,0.,150.));
#25517=CARTESIAN_POINT('',(89.1143010705401,-33.1608405307998,150.));
#25518=CARTESIAN_POINT('',(89.1143010705401,-33.1608405307998,150.));
#25519=CARTESIAN_POINT('',(90.3503690480399,-29.3566144656191,150.));
#25520=CARTESIAN_POINT('',(90.3503690480399,-29.3566144656191,150.));
#25521=CARTESIAN_POINT('',(90.3503690480399,-29.3566144656191,150.));
#25522=CARTESIAN_POINT('',(155.786207421713,8.16440917390091,150.));
#25523=CARTESIAN_POINT('',(159.780725560732,8.37375299887273,150.));
#25524=CARTESIAN_POINT('',(149.552104371408,44.3865754263987,150.));
#25525=CARTESIAN_POINT('Origin',(0.,0.,150.));
#25526=CARTESIAN_POINT('',(91.5864370255391,25.5523884004404,150.));
#25527=CARTESIAN_POINT('',(91.5864370255391,25.5523884004404,150.));
#25528=CARTESIAN_POINT('',(90.3503690480393,29.356614465621,150.));
#25529=CARTESIAN_POINT('',(90.3503690480393,29.356614465621,150.));
#25530=CARTESIAN_POINT('',(90.3503690480393,29.356614465621,150.));
#25531=CARTESIAN_POINT('',(3.,12.3,150.));
#25532=CARTESIAN_POINT('',(3.,-7.91840766518671E-16,150.));
#25533=CARTESIAN_POINT('',(-3.,12.3,150.));
#25534=CARTESIAN_POINT('',(-3.,-7.91840766518671E-16,150.));
#25535=CARTESIAN_POINT('',(0.,12.3,150.));
#25536=CARTESIAN_POINT('Origin',(0.,0.,0.));
#25537=CARTESIAN_POINT('',(3.,12.3,0.));
#25538=CARTESIAN_POINT('',(3.,12.3,0.));
#25539=CARTESIAN_POINT('',(-3.,12.3,0.));
#25540=CARTESIAN_POINT('',(3.,12.3,0.));
#25541=CARTESIAN_POINT('',(-3.,12.3,0.));
#25542=CARTESIAN_POINT('Origin',(0.,0.,87.5));
#25543=CARTESIAN_POINT('Origin',(0.,0.,137.5));
#25544=CARTESIAN_POINT('Origin',(0.,95.,330.));
#25545=CARTESIAN_POINT('',(4.,95.,320.));
#25546=CARTESIAN_POINT('',(4.,95.,330.));
#25547=CARTESIAN_POINT('',(0.,95.,320.));
#25548=CARTESIAN_POINT('',(0.,95.,320.));
#25549=CARTESIAN_POINT('',(0.,95.,330.));
#25550=CARTESIAN_POINT('Origin',(4.,95.,330.));
#25551=CARTESIAN_POINT('Origin',(4.,105.,320.));
#25552=CARTESIAN_POINT('',(4.00000000000002,155.948709516943,330.));
#25553=CARTESIAN_POINT('',(4.00000000000002,155.948709516943,330.));
#25554=CARTESIAN_POINT('',(4.,95.,330.));
#25555=CARTESIAN_POINT('Origin',(0.,0.,330.));
#25556=CARTESIAN_POINT('',(40.3757710359933,150.684428901095,330.));
#25557=CARTESIAN_POINT('',(40.3757710359933,150.684428901095,330.));
#25558=CARTESIAN_POINT('Origin',(0.,0.,330.));
#25559=CARTESIAN_POINT('Origin',(41.4110472164034,154.548132206251,330.));
#25560=CARTESIAN_POINT('',(41.4110472164034,154.548132206251,330.));
#25561=CARTESIAN_POINT('Origin',(0.,95.,330.));
#25562=CARTESIAN_POINT('Origin',(0.,105.,320.));
#25563=CARTESIAN_POINT('',(0.,95.,330.));
#25564=CARTESIAN_POINT('Origin',(0.,105.,320.));
#25565=CARTESIAN_POINT('Origin',(-55.8395989677851,76.85661446562,330.));
#25566=CARTESIAN_POINT('',(-52.6035309902853,79.2077554747898,320.));
#25567=CARTESIAN_POINT('',(-52.6035309902853,79.2077554747898,330.));
#25568=CARTESIAN_POINT('',(-55.8395989677851,76.85661446562,320.));
#25569=CARTESIAN_POINT('',(-55.8395989677851,76.85661446562,320.));
#25570=CARTESIAN_POINT('',(-55.8395989677851,76.85661446562,330.));
#25571=CARTESIAN_POINT('Origin',(-52.6035309902853,79.2077554747898,330.));
#25572=CARTESIAN_POINT('Origin',(-58.48138351321,87.2979254185393,320.));
#25573=CARTESIAN_POINT('',(-88.4282835906026,128.516297259219,330.));
#25574=CARTESIAN_POINT('',(-88.4282835906026,128.516297259219,330.));
#25575=CARTESIAN_POINT('',(-52.6035309902853,79.2077554747898,330.));
#25576=CARTESIAN_POINT('Origin',(0.,0.,330.));
#25577=CARTESIAN_POINT('',(-55.905400129067,145.638546533563,330.));
#25578=CARTESIAN_POINT('',(-55.905400129067,145.638546533563,330.));
#25579=CARTESIAN_POINT('Origin',(0.,0.,330.));
#25580=CARTESIAN_POINT('Origin',(-57.3388719272482,149.372868239552,330.));
#25581=CARTESIAN_POINT('',(-57.3388719272482,149.372868239552,330.));
#25582=CARTESIAN_POINT('Origin',(-55.8395989677851,76.85661446562,330.));
#25583=CARTESIAN_POINT('Origin',(-61.7174514907098,84.9467844093694,320.));
#25584=CARTESIAN_POINT('',(-55.8395989677851,76.85661446562,330.));
#25585=CARTESIAN_POINT('Origin',(-90.3503690480397,29.3566144656198,330.));
#25586=CARTESIAN_POINT('',(-89.1143010705399,33.1608405308004,320.));
#25587=CARTESIAN_POINT('',(-89.1143010705399,33.1608405308004,330.));
#25588=CARTESIAN_POINT('',(-90.3503690480397,29.3566144656198,320.));
#25589=CARTESIAN_POINT('',(-90.3503690480397,29.3566144656198,320.));
#25590=CARTESIAN_POINT('',(-90.3503690480397,29.3566144656198,330.));
#25591=CARTESIAN_POINT('Origin',(-89.1143010705399,33.1608405308004,330.));
#25592=CARTESIAN_POINT('Origin',(-98.6248662334914,36.2510104745498,320.));
#25593=CARTESIAN_POINT('',(-147.079968416409,51.9950275567578,330.));
#25594=CARTESIAN_POINT('',(-147.079968416409,51.9950275567578,330.));
#25595=CARTESIAN_POINT('',(-89.1143010705399,33.1608405308004,330.));
#25596=CARTESIAN_POINT('Origin',(0.,0.,330.));
#25597=CARTESIAN_POINT('',(-130.832608599486,84.963689462344,330.));
#25598=CARTESIAN_POINT('',(-130.832608599486,84.963689462344,330.));
#25599=CARTESIAN_POINT('Origin',(0.,0.,330.));
#25600=CARTESIAN_POINT('Origin',(-134.187290871268,87.142245602404,330.));
#25601=CARTESIAN_POINT('',(-134.187290871268,87.142245602404,330.));
#25602=CARTESIAN_POINT('Origin',(-90.3503690480397,29.3566144656198,330.));
#25603=CARTESIAN_POINT('Origin',(-99.8609342109912,32.4467844093692,320.));
#25604=CARTESIAN_POINT('',(-90.3503690480397,29.3566144656198,330.));
#25605=CARTESIAN_POINT('Origin',(-90.3503690480395,-29.3566144656204,330.));
#25606=CARTESIAN_POINT('',(-91.5864370255393,-25.5523884004398,320.));
#25607=CARTESIAN_POINT('',(-91.5864370255393,-25.5523884004398,330.));
#25608=CARTESIAN_POINT('',(-90.3503690480395,-29.3566144656204,320.));
#25609=CARTESIAN_POINT('',(-90.3503690480395,-29.3566144656204,320.));
#25610=CARTESIAN_POINT('',(-90.3503690480395,-29.3566144656204,330.));
#25611=CARTESIAN_POINT('Origin',(-91.5864370255393,-25.5523884004398,330.));
#25612=CARTESIAN_POINT('Origin',(-101.097002188491,-28.6425583441893,320.));
#25613=CARTESIAN_POINT('',(-149.552104371409,-44.3865754263977,330.));
#25614=CARTESIAN_POINT('',(-149.552104371409,-44.3865754263977,330.));
#25615=CARTESIAN_POINT('',(-91.5864370255393,-25.5523884004398,330.));
#25616=CARTESIAN_POINT('Origin',(0.,0.,330.));
#25617=CARTESIAN_POINT('',(-155.786207421714,-8.16440917389982,330.));
#25618=CARTESIAN_POINT('',(-155.786207421714,-8.16440917389982,330.));
#25619=CARTESIAN_POINT('Origin',(0.,0.,330.));
#25620=CARTESIAN_POINT('Origin',(-159.780725560732,-8.37375299887161,330.));
#25621=CARTESIAN_POINT('',(-159.780725560732,-8.37375299887161,330.));
#25622=CARTESIAN_POINT('Origin',(-90.3503690480395,-29.3566144656204,330.));
#25623=CARTESIAN_POINT('Origin',(-99.860934210991,-32.4467844093699,320.));
#25624=CARTESIAN_POINT('',(-90.3503690480395,-29.3566144656204,330.));
#25625=CARTESIAN_POINT('Origin',(-55.8395989677845,-76.8566144656203,330.));
#25626=CARTESIAN_POINT('',(-59.0756669452843,-74.5054734564505,320.));
#25627=CARTESIAN_POINT('',(-59.0756669452843,-74.5054734564505,330.));
#25628=CARTESIAN_POINT('',(-55.8395989677845,-76.8566144656203,320.));
#25629=CARTESIAN_POINT('',(-55.8395989677845,-76.8566144656203,320.));
#25630=CARTESIAN_POINT('',(-55.8395989677845,-76.8566144656203,330.));
#25631=CARTESIAN_POINT('Origin',(-59.0756669452843,-74.5054734564505,330.));
#25632=CARTESIAN_POINT('Origin',(-64.953519468209,-82.5956434001999,320.));
#25633=CARTESIAN_POINT('',(-94.9004195456013,-123.81401524088,330.));
#25634=CARTESIAN_POINT('',(-94.9004195456013,-123.81401524088,330.));
#25635=CARTESIAN_POINT('',(-59.0756669452843,-74.5054734564505,330.));
#25636=CARTESIAN_POINT('Origin',(0.,0.,330.));
#25637=CARTESIAN_POINT('',(-121.234769987287,-98.1739810037753,330.));
#25638=CARTESIAN_POINT('',(-121.234769987287,-98.1739810037753,330.));
#25639=CARTESIAN_POINT('Origin',(0.,0.,330.));
#25640=CARTESIAN_POINT('Origin',(-124.343353833115,-100.691262567975,330.));
#25641=CARTESIAN_POINT('',(-124.343353833115,-100.691262567975,330.));
#25642=CARTESIAN_POINT('Origin',(-55.8395989677845,-76.8566144656203,330.));
#25643=CARTESIAN_POINT('Origin',(-61.7174514907092,-84.9467844093698,320.));
#25644=CARTESIAN_POINT('',(-55.8395989677845,-76.8566144656203,330.));
#25645=CARTESIAN_POINT('Origin',(0.,-95.,330.));
#25646=CARTESIAN_POINT('',(-4.,-95.,320.));
#25647=CARTESIAN_POINT('',(-4.,-95.,330.));
#25648=CARTESIAN_POINT('',(0.,-95.,320.));
#25649=CARTESIAN_POINT('',(0.,-95.,320.));
#25650=CARTESIAN_POINT('',(0.,-95.,330.));
#25651=CARTESIAN_POINT('Origin',(-4.,-95.,330.));
#25652=CARTESIAN_POINT('Origin',(-4.,-105.,320.));
#25653=CARTESIAN_POINT('',(-4.00000000000002,-155.948709516943,330.));
#25654=CARTESIAN_POINT('',(-4.00000000000002,-155.948709516943,330.));
#25655=CARTESIAN_POINT('',(-4.,-95.,330.));
#25656=CARTESIAN_POINT('Origin',(0.,0.,330.));
#25657=CARTESIAN_POINT('',(-40.3757710359933,-150.684428901095,330.));
#25658=CARTESIAN_POINT('',(-40.3757710359933,-150.684428901095,330.));
#25659=CARTESIAN_POINT('Origin',(0.,0.,330.));
#25660=CARTESIAN_POINT('Origin',(-41.4110472164034,-154.548132206251,330.));
#25661=CARTESIAN_POINT('',(-41.4110472164034,-154.548132206251,330.));
#25662=CARTESIAN_POINT('Origin',(0.,-95.,330.));
#25663=CARTESIAN_POINT('Origin',(0.,-105.,320.));
#25664=CARTESIAN_POINT('',(0.,-95.,330.));
#25665=CARTESIAN_POINT('Origin',(55.8395989677856,-76.8566144656195,330.));
#25666=CARTESIAN_POINT('',(52.6035309902859,-79.2077554747894,320.));
#25667=CARTESIAN_POINT('',(52.6035309902859,-79.2077554747894,330.));
#25668=CARTESIAN_POINT('',(55.8395989677856,-76.8566144656195,320.));
#25669=CARTESIAN_POINT('',(55.8395989677856,-76.8566144656195,320.));
#25670=CARTESIAN_POINT('',(55.8395989677856,-76.8566144656195,330.));
#25671=CARTESIAN_POINT('Origin',(52.6035309902859,-79.2077554747894,330.));
#25672=CARTESIAN_POINT('Origin',(58.4813835132107,-87.2979254185389,320.));
#25673=CARTESIAN_POINT('',(88.4282835906035,-128.516297259218,330.));
#25674=CARTESIAN_POINT('',(88.4282835906035,-128.516297259218,330.));
#25675=CARTESIAN_POINT('',(52.6035309902859,-79.2077554747894,330.));
#25676=CARTESIAN_POINT('Origin',(0.,0.,330.));
#25677=CARTESIAN_POINT('',(55.905400129068,-145.638546533563,330.));
#25678=CARTESIAN_POINT('',(55.905400129068,-145.638546533563,330.));
#25679=CARTESIAN_POINT('Origin',(0.,0.,330.));
#25680=CARTESIAN_POINT('Origin',(57.3388719272493,-149.372868239552,330.));
#25681=CARTESIAN_POINT('',(57.3388719272493,-149.372868239552,330.));
#25682=CARTESIAN_POINT('Origin',(55.8395989677856,-76.8566144656195,330.));
#25683=CARTESIAN_POINT('Origin',(61.7174514907104,-84.9467844093689,320.));
#25684=CARTESIAN_POINT('',(55.8395989677856,-76.8566144656195,330.));
#25685=CARTESIAN_POINT('Origin',(90.3503690480399,-29.3566144656191,330.));
#25686=CARTESIAN_POINT('',(89.1143010705401,-33.1608405307998,320.));
#25687=CARTESIAN_POINT('',(89.1143010705401,-33.1608405307998,330.));
#25688=CARTESIAN_POINT('',(90.3503690480399,-29.3566144656191,320.));
#25689=CARTESIAN_POINT('',(90.3503690480399,-29.3566144656191,320.));
#25690=CARTESIAN_POINT('',(90.3503690480399,-29.3566144656191,330.));
#25691=CARTESIAN_POINT('Origin',(89.1143010705401,-33.1608405307998,330.));
#25692=CARTESIAN_POINT('Origin',(98.6248662334917,-36.2510104745491,320.));
#25693=CARTESIAN_POINT('',(147.07996841641,-51.9950275567568,330.));
#25694=CARTESIAN_POINT('',(147.07996841641,-51.9950275567568,330.));
#25695=CARTESIAN_POINT('',(89.1143010705401,-33.1608405307998,330.));
#25696=CARTESIAN_POINT('Origin',(0.,0.,330.));
#25697=CARTESIAN_POINT('',(130.832608599487,-84.9636894623431,330.));
#25698=CARTESIAN_POINT('',(130.832608599487,-84.9636894623431,330.));
#25699=CARTESIAN_POINT('Origin',(0.,0.,330.));
#25700=CARTESIAN_POINT('Origin',(134.187290871269,-87.1422456024031,330.));
#25701=CARTESIAN_POINT('',(134.187290871269,-87.1422456024031,330.));
#25702=CARTESIAN_POINT('Origin',(90.3503690480399,-29.3566144656191,330.));
#25703=CARTESIAN_POINT('Origin',(99.8609342109914,-32.4467844093685,320.));
#25704=CARTESIAN_POINT('',(90.3503690480399,-29.3566144656191,330.));
#25705=CARTESIAN_POINT('Origin',(90.3503690480393,29.356614465621,330.));
#25706=CARTESIAN_POINT('',(91.5864370255391,25.5523884004404,320.));
#25707=CARTESIAN_POINT('',(91.5864370255391,25.5523884004404,330.));
#25708=CARTESIAN_POINT('',(90.3503690480393,29.356614465621,320.));
#25709=CARTESIAN_POINT('',(90.3503690480393,29.356614465621,320.));
#25710=CARTESIAN_POINT('',(90.3503690480393,29.356614465621,330.));
#25711=CARTESIAN_POINT('Origin',(91.5864370255391,25.5523884004404,330.));
#25712=CARTESIAN_POINT('Origin',(101.097002188491,28.64255834419,320.));
#25713=CARTESIAN_POINT('',(149.552104371408,44.3865754263987,330.));
#25714=CARTESIAN_POINT('',(149.552104371408,44.3865754263987,330.));
#25715=CARTESIAN_POINT('',(91.5864370255391,25.5523884004404,330.));
#25716=CARTESIAN_POINT('Origin',(0.,0.,330.));
#25717=CARTESIAN_POINT('',(155.786207421713,8.16440917390091,330.));
#25718=CARTESIAN_POINT('',(155.786207421713,8.16440917390091,330.));
#25719=CARTESIAN_POINT('Origin',(0.,0.,330.));
#25720=CARTESIAN_POINT('Origin',(159.780725560732,8.37375299887273,330.));
#25721=CARTESIAN_POINT('',(159.780725560732,8.37375299887273,330.));
#25722=CARTESIAN_POINT('Origin',(90.3503690480393,29.356614465621,330.));
#25723=CARTESIAN_POINT('Origin',(99.8609342109908,32.4467844093706,320.));
#25724=CARTESIAN_POINT('',(90.3503690480393,29.356614465621,330.));
#25725=CARTESIAN_POINT('Origin',(55.8395989677839,76.8566144656207,330.));
#25726=CARTESIAN_POINT('',(59.0756669452838,74.5054734564509,320.));
#25727=CARTESIAN_POINT('',(59.0756669452838,74.5054734564509,330.));
#25728=CARTESIAN_POINT('',(55.8395989677839,76.8566144656207,320.));
#25729=CARTESIAN_POINT('',(55.8395989677839,76.8566144656207,320.));
#25730=CARTESIAN_POINT('',(55.8395989677839,76.8566144656207,330.));
#25731=CARTESIAN_POINT('Origin',(59.0756669452838,74.5054734564509,330.));
#25732=CARTESIAN_POINT('Origin',(64.9535194682084,82.5956434002004,320.));
#25733=CARTESIAN_POINT('',(94.9004195456004,123.814015240881,330.));
#25734=CARTESIAN_POINT('',(94.9004195456004,123.814015240881,330.));
#25735=CARTESIAN_POINT('',(59.0756669452838,74.5054734564509,330.));
#25736=CARTESIAN_POINT('Origin',(0.,0.,330.));
#25737=CARTESIAN_POINT('',(121.234769987286,98.1739810037762,330.));
#25738=CARTESIAN_POINT('',(121.234769987286,98.1739810037762,330.));
#25739=CARTESIAN_POINT('Origin',(0.,0.,330.));
#25740=CARTESIAN_POINT('Origin',(124.343353833114,100.691262567976,330.));
#25741=CARTESIAN_POINT('',(124.343353833114,100.691262567976,330.));
#25742=CARTESIAN_POINT('Origin',(55.8395989677839,76.8566144656207,330.));
#25743=CARTESIAN_POINT('Origin',(61.7174514907085,84.9467844093703,320.));
#25744=CARTESIAN_POINT('',(55.8395989677839,76.8566144656207,330.));
#25745=CARTESIAN_POINT('Origin',(-61.7174514907098,84.9467844093694,320.));
#25746=CARTESIAN_POINT('Origin',(-99.8609342109912,32.4467844093692,320.));
#25747=CARTESIAN_POINT('Origin',(-99.860934210991,-32.4467844093699,320.));
#25748=CARTESIAN_POINT('Origin',(-61.7174514907092,-84.9467844093698,320.));
#25749=CARTESIAN_POINT('Origin',(0.,-105.,320.));
#25750=CARTESIAN_POINT('Origin',(61.7174514907104,-84.9467844093689,320.));
#25751=CARTESIAN_POINT('Origin',(99.8609342109914,-32.4467844093685,320.));
#25752=CARTESIAN_POINT('Origin',(99.8609342109908,32.4467844093706,320.));
#25753=CARTESIAN_POINT('Origin',(61.7174514907085,84.9467844093703,320.));
#25754=CARTESIAN_POINT('Origin',(0.,0.,330.));
#25755=CARTESIAN_POINT('Origin',(0.,0.,330.));
#25756=CARTESIAN_POINT('Origin',(0.,0.,330.));
#25757=CARTESIAN_POINT('Origin',(0.,0.,330.));
#25758=CARTESIAN_POINT('Origin',(0.,0.,330.));
#25759=CARTESIAN_POINT('Origin',(0.,0.,330.));
#25760=CARTESIAN_POINT('Origin',(0.,0.,330.));
#25761=CARTESIAN_POINT('Origin',(0.,0.,330.));
#25762=CARTESIAN_POINT('Origin',(0.,0.,330.));
#25763=CARTESIAN_POINT('Origin',(0.,0.,330.));
#25764=CARTESIAN_POINT('Origin',(0.,0.,342.5));
#25765=CARTESIAN_POINT('Origin',(3.,12.3,342.5));
#25766=CARTESIAN_POINT('',(3.,12.3,342.5));
#25767=CARTESIAN_POINT('Origin',(3.,12.3,342.5));
#25768=CARTESIAN_POINT('',(-3.,12.3,342.5));
#25769=CARTESIAN_POINT('Origin',(-3.,12.3,342.5));
#27532=UNCERTAINTY_MEASURE_WITH_UNIT(LENGTH_MEASURE(0.01),#27542,
'DISTANCE_ACCURACY_VALUE',
'Maximum model space distance between geometric entities at asserted c
onnectivities');
#27535=UNCERTAINTY_MEASURE_WITH_UNIT(LENGTH_MEASURE(0.01),#27542,
'DISTANCE_ACCURACY_VALUE',
'Maximum model space distance between geometric entities at asserted c
onnectivities');
#27538=(
GEOMETRIC_REPRESENTATION_CONTEXT(3)
GLOBAL_UNCERTAINTY_ASSIGNED_CONTEXT((#27532))
GLOBAL_UNIT_ASSIGNED_CONTEXT((#27542,#27544,#27545))
REPRESENTATION_CONTEXT('','3D')
);
#27541=(
GEOMETRIC_REPRESENTATION_CONTEXT(3)
GLOBAL_UNCERTAINTY_ASSIGNED_CONTEXT((#27535))
GLOBAL_UNIT_ASSIGNED_CONTEXT((#27542,#27544,#27545))
REPRESENTATION_CONTEXT('','3D')
);
#27542=(
LENGTH_UNIT()
NAMED_UNIT(*)
SI_UNIT(.MILLI.,.METRE.)
);
#27544=(
NAMED_UNIT(*)
PLANE_ANGLE_UNIT()
SI_UNIT($,.RADIAN.)
);
#27545=(
NAMED_UNIT(*)
SI_UNIT($,.STERADIAN.)
SOLID_ANGLE_UNIT()
);
#27548=SHAPE_DEFINITION_REPRESENTATION(#27553,#27562);
#27553=PRODUCT_DEFINITION_SHAPE('',$,#27568);
#27562=SHAPE_REPRESENTATION('',(#12424),#27538);
#27565=PRODUCT_DEFINITION_CONTEXT('part definition',#27582,'design');
#27568=PRODUCT_DEFINITION('2. Impeller','2. Impeller',#27573,#27565);
#27573=PRODUCT_DEFINITION_FORMATION('',$,#27586);
#27582=APPLICATION_CONTEXT(
'Core Data for Automotive Mechanical Design Process');
#27583=PRODUCT_CONTEXT('part definition',#27582,'mechanical');
#27586=PRODUCT('2. Impeller','2. Impeller',$,(#27583));
#27591=PRESENTATION_STYLE_ASSIGNMENT((#27595));
#27595=SURFACE_STYLE_USAGE(.BOTH.,#27599);
#27599=SURFACE_SIDE_STYLE('',(#27603));
#27603=SURFACE_STYLE_FILL_AREA(#27607);
#27607=FILL_AREA_STYLE('Opaque(227,224,212)',(#27611));
#27611=FILL_AREA_STYLE_COLOUR('Opaque(227,224,212)',#27615);
#27615=COLOUR_RGB('Opaque(227,224,212)',0.890196078431372,0.87843137254902,
0.831372549019608);
ENDSEC;
END-ISO-10303-21;
